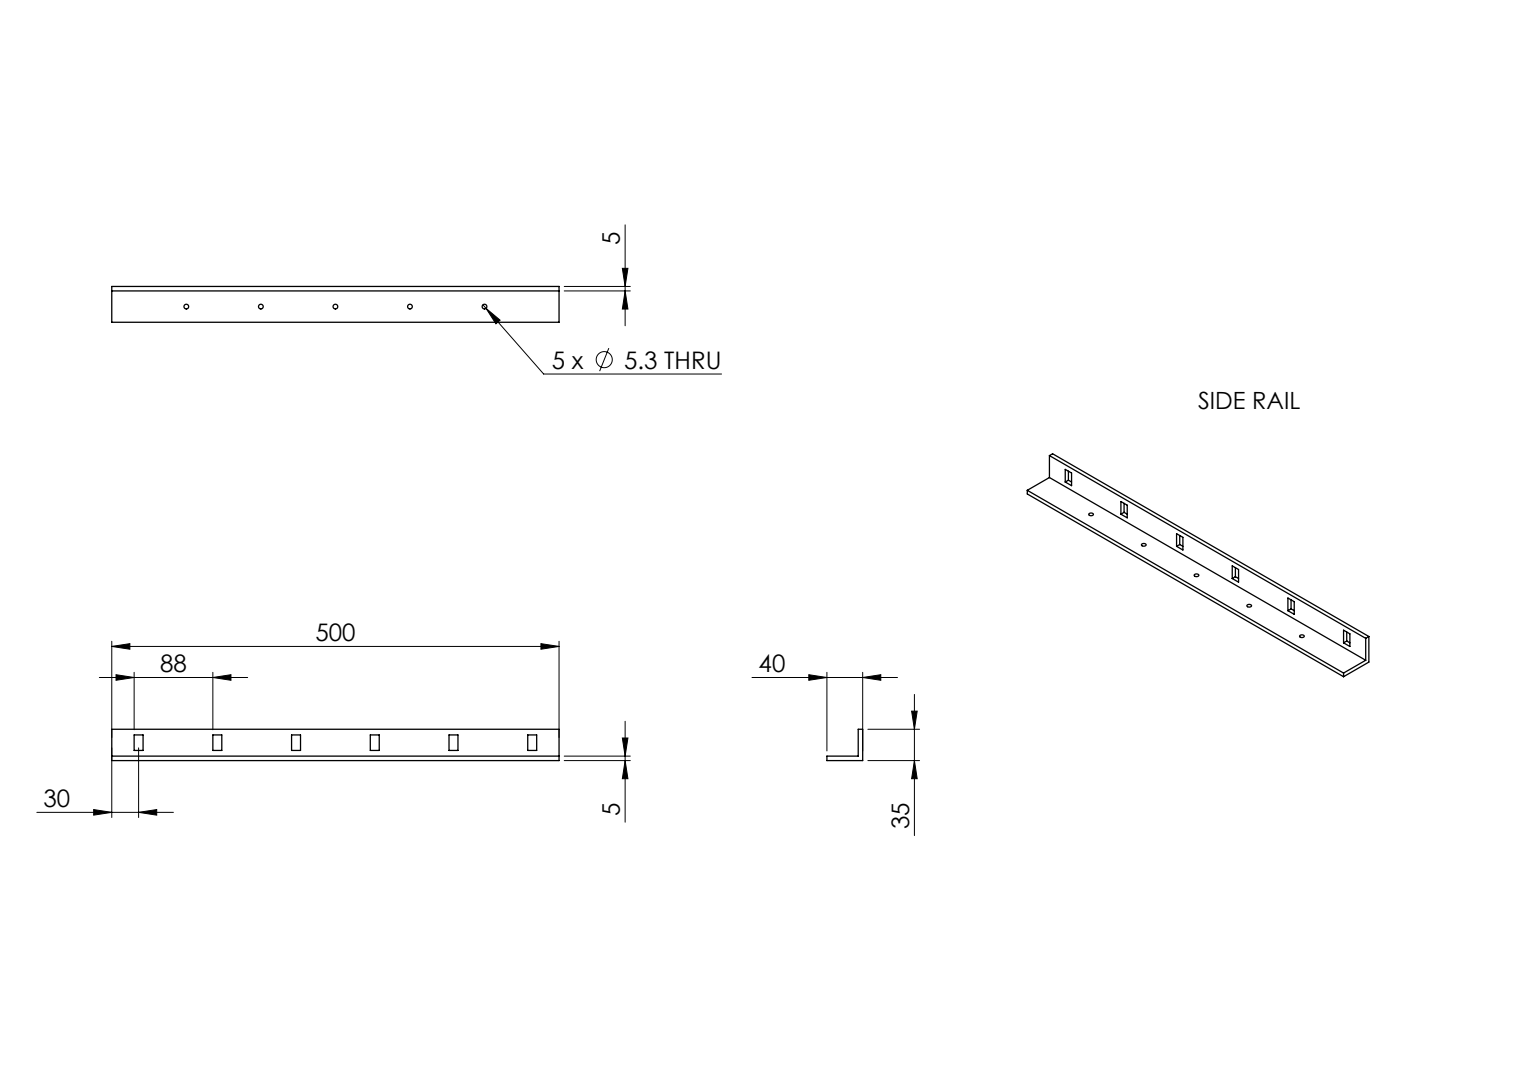
ISO-10303-21;
HEADER;
FILE_DESCRIPTION (('STEP AP214'),
    '1' );
FILE_NAME ('side rail.step',
    '2026-10-24T13:33:06',
    ( '' ),
    ( '' ),
    'SwSTEP 2.0',
    'SolidWorks 2026',
    '' );
FILE_SCHEMA (( 'AUTOMOTIVE_DESIGN' ));
ENDSEC;

DATA;
#21=VECTOR ( 'NONE', #6060, 1000.000000000000000 ) ;
#37=ADVANCED_FACE ( 'NONE', ( #11695 ), #12926, .T. ) ;
#81=ADVANCED_FACE ( 'NONE', ( #7413, #11845, #1899, #419, #4888, #9306, #3544 ), #4372, .T. ) ;
#89=PLANE ( 'NONE',  #11765 ) ;
#114=ORIENTED_EDGE ( 'NONE', *, *, #1574, .F. ) ;
#116=AXIS2_PLACEMENT_3D ( 'NONE', #1990, #12809, #3959 ) ;
#129=CARTESIAN_POINT ( 'NONE',  ( 357.0000000000000000, 8.660254037844390851, 205.0000000000000284 ) ) ;
#143=CARTESIAN_POINT ( 'NONE',  ( 93.00000000000000000, -8.660254037844389075, 199.9990000000000236 ) ) ;
#156=ADVANCED_FACE ( 'NONE', ( #2113 ), #8789, .F. ) ;
#158=CYLINDRICAL_SURFACE ( 'NONE', #4474, 2.649999999999985700 ) ;
#167=EDGE_CURVE ( 'NONE', #11965, #7113, #13067, .T. ) ;
#176=DIRECTION ( 'NONE',  ( -0.000000000000000000, 1.000000000000000000, 0.000000000000000000 ) ) ;
#194=DIRECTION ( 'NONE',  ( 1.000000000000000000, 0.000000000000000000, 0.000000000000000000 ) ) ;
#222=VECTOR ( 'NONE', #1616, 1000.000000000000000 ) ;
#227=FILL_AREA_STYLE ('',( #2582 ) ) ;
#231=LINE ( 'NONE', #7733, #9690 ) ;
#254=DIRECTION ( 'NONE',  ( -1.000000000000000000, 0.000000000000000000, 0.000000000000000000 ) ) ;
#257=ORIENTED_EDGE ( 'NONE', *, *, #9709, .T. ) ;
#259=DIRECTION ( 'NONE',  ( 0.000000000000000000, 0.000000000000000000, 1.000000000000000000 ) ) ;
#261=ORIENTED_EDGE ( 'NONE', *, *, #3754, .T. ) ;
#280=EDGE_LOOP ( 'NONE', ( #548, #583, #6220, #3150 ) ) ;
#285=CARTESIAN_POINT ( 'NONE',  ( 259.0000000000000000, 8.660254037844390851, 205.0000000000000284 ) ) ;
#302=EDGE_CURVE ( 'NONE', #5376, #611, #2399, .T. ) ;
#303=FACE_OUTER_BOUND ( 'NONE', #3913, .T. ) ;
#308=EDGE_CURVE ( 'NONE', #574, #7171, #11477, .T. ) ;
#311=DIRECTION ( 'NONE',  ( -0.000000000000000000, 1.000000000000000000, 0.000000000000000000 ) ) ;
#327=ADVANCED_FACE ( 'NONE', ( #11322 ), #1364, .F. ) ;
#335=DIRECTION ( 'NONE',  ( 0.000000000000000000, 1.000000000000000000, 0.000000000000000000 ) ) ;
#340=EDGE_CURVE ( 'NONE', #10091, #12864, #5804, .T. ) ;
#352=EDGE_LOOP ( 'NONE', ( #7551, #6628 ) ) ;
#359=VECTOR ( 'NONE', #3088, 1000.000000000000000 ) ;
#373=CIRCLE ( 'NONE', #6200, 2.649999999999985700 ) ;
#392=VECTOR ( 'NONE', #9688, 1000.000000000000000 ) ;
#393=DIRECTION ( 'NONE',  ( 0.000000000000000000, 0.000000000000000000, 1.000000000000000000 ) ) ;
#396=ORIENTED_EDGE ( 'NONE', *, *, #10733, .F. ) ;
#397=CARTESIAN_POINT ( 'NONE',  ( 82.99999999999998579, -8.660254037844389075, 200.0000000000000000 ) ) ;
#410=CARTESIAN_POINT ( 'NONE',  ( -30.00000000000002842, 15.00000000000000000, 205.0000000000000284 ) ) ;
#419=FACE_BOUND ( 'NONE', #9154, .T. ) ;
#424=ORIENTED_EDGE ( 'NONE', *, *, #1321, .T. ) ;
#426=ADVANCED_FACE ( 'NONE', ( #13912 ), #3987, .F. ) ;
#427=DIRECTION ( 'NONE',  ( -1.000000000000000000, 0.000000000000000000, 0.000000000000000000 ) ) ;
#441=LINE ( 'NONE', #4910, #14145 ) ;
#471=VECTOR ( 'NONE', #1834, 1000.000000000000000 ) ;
#486=VERTEX_POINT ( 'NONE', #1503 ) ;
#487=FACE_BOUND ( 'NONE', #5303, .T. ) ;
#494=DIRECTION ( 'NONE',  ( -0.000000000000000000, -0.000000000000000000, 1.000000000000000000 ) ) ;
#507=LINE ( 'NONE', #9385, #4377 ) ;
#514=VERTEX_POINT ( 'NONE', #397 ) ;
#515=( LENGTH_UNIT ( ) NAMED_UNIT ( * ) SI_UNIT ( .MILLI., .METRE. ) );
#521=ORIENTED_EDGE ( 'NONE', *, *, #4268, .F. ) ;
#526=VECTOR ( 'NONE', #13201, 1000.000000000000000 ) ;
#532=VERTEX_POINT ( 'NONE', #10807 ) ;
#537=CARTESIAN_POINT ( 'NONE',  ( 347.0000000000000000, 8.660254037844390851, 199.9990000000000236 ) ) ;
#544=AXIS2_PLACEMENT_3D ( 'NONE', #926, #9879, #13212 ) ;
#545=DIRECTION ( 'NONE',  ( 0.000000000000000000, 0.000000000000000000, 1.000000000000000000 ) ) ;
#548=ORIENTED_EDGE ( 'NONE', *, *, #9525, .F. ) ;
#549=DIRECTION ( 'NONE',  ( -1.000000000000000000, 0.000000000000000000, -0.000000000000000000 ) ) ;
#554=DIRECTION ( 'NONE',  ( 0.000000000000000000, 0.000000000000000000, 1.000000000000000000 ) ) ;
#558=ORIENTED_EDGE ( 'NONE', *, *, #6357, .F. ) ;
#559=FACE_BOUND ( 'NONE', #6521, .T. ) ;
#560=ADVANCED_FACE ( 'NONE', ( #13188 ), #11821, .F. ) ;
#574=VERTEX_POINT ( 'NONE', #11897 ) ;
#583=ORIENTED_EDGE ( 'NONE', *, *, #10908, .F. ) ;
#590=LINE ( 'NONE', #1845, #7331 ) ;
#607=CARTESIAN_POINT ( 'NONE',  ( 53.33333333333330017, -20.00000000000000000, 225.1500000000000625 ) ) ;
#611=VERTEX_POINT ( 'NONE', #9793 ) ;
#617=DIRECTION ( 'NONE',  ( -0.000000000000000000, -0.000000000000000000, 1.000000000000000000 ) ) ;
#621=DIRECTION ( 'NONE',  ( -0.000000000000000000, -0.000000000000000000, 1.000000000000000000 ) ) ;
#622=FACE_BOUND ( 'NONE', #8043, .T. ) ;
#629=ORIENTED_EDGE ( 'NONE', *, *, #10325, .T. ) ;
#633=CARTESIAN_POINT ( 'NONE',  ( 386.6666666666666288, -14.99999999999999822, 219.8500000000001080 ) ) ;
#638=EDGE_LOOP ( 'NONE', ( #7545, #6355, #6179, #9350 ) ) ;
#643=ADVANCED_FACE ( 'NONE', ( #9643 ), #839, .F. ) ;
#696=ORIENTED_EDGE ( 'NONE', *, *, #2963, .T. ) ;
#703=PLANE ( 'NONE',  #2931 ) ;
#709=FACE_OUTER_BOUND ( 'NONE', #10738, .T. ) ;
#718=ORIENTED_EDGE ( 'NONE', *, *, #4541, .F. ) ;
#720=EDGE_CURVE ( 'NONE', #10091, #8663, #9863, .T. ) ;
#725=CARTESIAN_POINT ( 'NONE',  ( 259.0000000000000000, 8.660254037844390851, 199.9990000000000236 ) ) ;
#730=DIRECTION ( 'NONE',  ( 1.000000000000000000, 0.000000000000000000, 0.000000000000000000 ) ) ;
#744=ORIENTED_EDGE ( 'NONE', *, *, #9206, .T. ) ;
#769=LINE ( 'NONE', #1579, #4481 ) ;
#784=EDGE_LOOP ( 'NONE', ( #12621, #13135, #7197, #6469 ) ) ;
#788=AXIS2_PLACEMENT_3D ( 'NONE', #10096, #13425, #6557 ) ;
#792=ORIENTED_EDGE ( 'NONE', *, *, #4975, .T. ) ;
#797=CARTESIAN_POINT ( 'NONE',  ( 170.9999999999999716, -8.660254037844389075, 205.0000000000000284 ) ) ;
#806=VERTEX_POINT ( 'NONE', #6663 ) ;
#807=DIRECTION ( 'NONE',  ( 0.000000000000000000, -1.000000000000000000, 0.000000000000000000 ) ) ;
#808=CIRCLE ( 'NONE', #6622, 2.649999999999985700 ) ;
#822=EDGE_LOOP ( 'NONE', ( #3970, #8831, #13317, #6166 ) ) ;
#829=PRODUCT_DEFINITION_CONTEXT ( 'detailed design', #10547, 'design' ) ;
#830=ORIENTED_EDGE ( 'NONE', *, *, #8702, .T. ) ;
#831=DIRECTION ( 'NONE',  ( -0.000000000000000000, 1.000000000000000000, -0.000000000000000000 ) ) ;
#839=PLANE ( 'NONE',  #11489 ) ;
#855=DIRECTION ( 'NONE',  ( 1.000000000000000000, 0.000000000000000000, 0.000000000000000000 ) ) ;
#862=UNCERTAINTY_MEASURE_WITH_UNIT (LENGTH_MEASURE( 1.000000000000000082E-05 ), #515, 'distance_accuracy_value', 'NONE');
#876=AXIS2_PLACEMENT_3D ( 'NONE', #2252, #11112, #2107 ) ;
#898=VERTEX_POINT ( 'NONE', #607 ) ;
#900=EDGE_CURVE ( 'NONE', #7113, #7167, #1368, .T. ) ;
#906=ORIENTED_EDGE ( 'NONE', *, *, #9206, .F. ) ;
#913=FACE_OUTER_BOUND ( 'NONE', #14136, .T. ) ;
#917=CIRCLE ( 'NONE', #12520, 2.649999999999985700 ) ;
#920=FACE_OUTER_BOUND ( 'NONE', #822, .T. ) ;
#925=EDGE_LOOP ( 'NONE', ( #10023, #943, #257, #1375 ) ) ;
#926=CARTESIAN_POINT ( 'NONE',  ( 303.3333333333333144, -15.00000000000000000, 222.5000000000000853 ) ) ;
#930=VERTEX_POINT ( 'NONE', #2815 ) ;
#943=ORIENTED_EDGE ( 'NONE', *, *, #2678, .T. ) ;
#962=CARTESIAN_POINT ( 'NONE',  ( 82.99999999999998579, 8.660254037844390851, 205.0000000000000284 ) ) ;
#964=ORIENTED_EDGE ( 'NONE', *, *, #6331, .T. ) ;
#970=DIRECTION ( 'NONE',  ( 0.000000000000000000, -1.000000000000000000, 0.000000000000000000 ) ) ;
#994=LINE ( 'NONE', #9059, #12994 ) ;
#1021=ORIENTED_EDGE ( 'NONE', *, *, #11142, .T. ) ;
#1041=DIRECTION ( 'NONE',  ( -0.000000000000000000, 1.000000000000000000, 0.000000000000000000 ) ) ;
#1063=DIRECTION ( 'NONE',  ( 0.000000000000000000, 0.000000000000000000, -1.000000000000000000 ) ) ;
#1070=VECTOR ( 'NONE', #2045, 1000.000000000000000 ) ;
#1106=PLANE ( 'NONE',  #10917 ) ;
#1107=LINE ( 'NONE', #5555, #2077 ) ;
#1139=LINE ( 'NONE', #5516, #526 ) ;
#1151=VERTEX_POINT ( 'NONE', #8203 ) ;
#1155=EDGE_CURVE ( 'NONE', #12855, #4614, #1461, .T. ) ;
#1156=EDGE_LOOP ( 'NONE', ( #5436, #9530, #5592, #6967 ) ) ;
#1158=EDGE_LOOP ( 'NONE', ( #6888, #7499, #114, #558 ) ) ;
#1182=CARTESIAN_POINT ( 'NONE',  ( 136.6666666666666288, -20.00000000000000000, 222.5000000000000853 ) ) ;
#1209=ORIENTED_EDGE ( 'NONE', *, *, #1854, .T. ) ;
#1221=EDGE_CURVE ( 'NONE', #8720, #14065, #6982, .T. ) ;
#1227=LINE ( 'NONE', #3497, #6780 ) ;
#1228=ORIENTED_EDGE ( 'NONE', *, *, #5685, .F. ) ;
#1233=DIRECTION ( 'NONE',  ( 0.000000000000000000, 0.000000000000000000, 1.000000000000000000 ) ) ;
#1236=( NAMED_UNIT ( * ) SI_UNIT ( $, .STERADIAN. ) SOLID_ANGLE_UNIT ( ) );
#1250=EDGE_CURVE ( 'NONE', #4587, #12687, #13572, .T. ) ;
#1277=DIRECTION ( 'NONE',  ( 0.000000000000000000, -1.000000000000000000, 0.000000000000000000 ) ) ;
#1308=CARTESIAN_POINT ( 'NONE',  ( 303.3333333333333144, -15.00000000000000000, 225.1500000000000625 ) ) ;
#1321=EDGE_CURVE ( 'NONE', #13567, #5456, #13939, .T. ) ;
#1332=VERTEX_POINT ( 'NONE', #4961 ) ;
#1346=CARTESIAN_POINT ( 'NONE',  ( 386.6666666666666288, -20.00000000000000000, 222.5000000000000853 ) ) ;
#1350=EDGE_CURVE ( 'NONE', #5388, #6497, #3002, .T. ) ;
#1356=FACE_OUTER_BOUND ( 'NONE', #5395, .T. ) ;
#1364=CYLINDRICAL_SURFACE ( 'NONE', #3147, 2.649999999999985700 ) ;
#1366=CARTESIAN_POINT ( 'NONE',  ( 434.9999999999999432, 8.660254037844390851, 199.9990000000000236 ) ) ;
#1368=CIRCLE ( 'NONE', #12741, 2.649999999999985700 ) ;
#1375=ORIENTED_EDGE ( 'NONE', *, *, #13935, .T. ) ;
#1393=VECTOR ( 'NONE', #7157, 1000.000000000000000 ) ;
#1423=EDGE_LOOP ( 'NONE', ( #8180, #5861, #11249, #6169 ) ) ;
#1426=CARTESIAN_POINT ( 'NONE',  ( 434.9999999999999432, -8.660254037844389075, 199.9990000000000236 ) ) ;
#1445=VECTOR ( 'NONE', #3310, 1000.000000000000000 ) ;
#1461=LINE ( 'NONE', #5971, #12295 ) ;
#1462=EDGE_LOOP ( 'NONE', ( #7055, #3073, #3390, #9366, #2015, #2649 ) ) ;
#1472=ORIENTED_EDGE ( 'NONE', *, *, #302, .F. ) ;
#1476=CARTESIAN_POINT ( 'NONE',  ( 181.0000000000000000, 8.660254037844390851, 200.0000000000000000 ) ) ;
#1496=ADVANCED_FACE ( 'NONE', ( #10029 ), #9955, .F. ) ;
#1500=ORIENTED_EDGE ( 'NONE', *, *, #7562, .F. ) ;
#1503=CARTESIAN_POINT ( 'NONE',  ( 93.00000000000000000, 8.660254037844390851, 200.0000000000000000 ) ) ;
#1511=DIRECTION ( 'NONE',  ( 1.000000000000000000, 0.000000000000000000, 0.000000000000000000 ) ) ;
#1521=VECTOR ( 'NONE', #4856, 1000.000000000000000 ) ;
#1525=EDGE_LOOP ( 'NONE', ( #12096, #1587 ) ) ;
#1533=ORIENTED_EDGE ( 'NONE', *, *, #302, .T. ) ;
#1534=CARTESIAN_POINT ( 'NONE',  ( -5.000000000000000888, 8.660254037844390851, 205.0000000000000284 ) ) ;
#1543=VECTOR ( 'NONE', #13285, 1000.000000000000000 ) ;
#1544=ORIENTED_EDGE ( 'NONE', *, *, #720, .F. ) ;
#1547=DIRECTION ( 'NONE',  ( 0.000000000000000000, 0.000000000000000000, 1.000000000000000000 ) ) ;
#1553=EDGE_CURVE ( 'NONE', #8456, #8038, #4796, .T. ) ;
#1574=EDGE_CURVE ( 'NONE', #3366, #4058, #6753, .T. ) ;
#1576=EDGE_CURVE ( 'NONE', #8786, #486, #1227, .T. ) ;
#1579=CARTESIAN_POINT ( 'NONE',  ( 470.0000000000000000, 15.00000000000000000, 205.0000000000000284 ) ) ;
#1586=DIRECTION ( 'NONE',  ( 1.000000000000000000, 0.000000000000000000, 0.000000000000000000 ) ) ;
#1587=ORIENTED_EDGE ( 'NONE', *, *, #6484, .T. ) ;
#1590=CARTESIAN_POINT ( 'NONE',  ( 259.0000000000000000, -8.660254037844389075, 200.0000000000000000 ) ) ;
#1606=LINE ( 'NONE', #4020, #8260 ) ;
#1616=DIRECTION ( 'NONE',  ( 0.000000000000000000, 1.000000000000000000, 0.000000000000000000 ) ) ;
#1650=ORIENTED_EDGE ( 'NONE', *, *, #13490, .T. ) ;
#1659=CARTESIAN_POINT ( 'NONE',  ( 136.6666666666666288, -14.99999999999999822, 219.8500000000001080 ) ) ;
#1661=VECTOR ( 'NONE', #6856, 1000.000000000000000 ) ;
#1673=EDGE_LOOP ( 'NONE', ( #9501, #13329, #5600, #2944 ) ) ;
#1675=CIRCLE ( 'NONE', #11651, 2.649999999999985700 ) ;
#1692=ORIENTED_EDGE ( 'NONE', *, *, #11438, .T. ) ;
#1698=ORIENTED_EDGE ( 'NONE', *, *, #11906, .T. ) ;
#1712=DIRECTION ( 'NONE',  ( 0.000000000000000000, -0.000000000000000000, -1.000000000000000000 ) ) ;
#1715=CARTESIAN_POINT ( 'NONE',  ( 434.9999999999999432, -8.660254037844389075, 205.0000000000000284 ) ) ;
#1732=CARTESIAN_POINT ( 'NONE',  ( 269.0000000000000000, -8.660254037844389075, 200.0000000000000000 ) ) ;
#1746=CARTESIAN_POINT ( 'NONE',  ( 269.0000000000000000, 8.660254037844390851, 205.0000000000000284 ) ) ;
#1757=CIRCLE ( 'NONE', #14043, 2.649999999999985700 ) ;
#1760=ADVANCED_BREP_SHAPE_REPRESENTATION ( '', ( #3714, #14039 ), #3087 ) ;
#1772=VECTOR ( 'NONE', #10843, 1000.000000000000000 ) ;
#1779=LINE ( 'NONE', #8531, #7857 ) ;
#1789=DIRECTION ( 'NONE',  ( -0.000000000000000000, -0.000000000000000000, 1.000000000000000000 ) ) ;
#1794=AXIS2_PLACEMENT_3D ( 'NONE', #11740, #10875, #9715 ) ;
#1797=EDGE_CURVE ( 'NONE', #2838, #12140, #769, .T. ) ;
#1822=EDGE_LOOP ( 'NONE', ( #13493, #1021, #5094, #2101 ) ) ;
#1834=DIRECTION ( 'NONE',  ( 0.000000000000000000, 1.000000000000000000, 0.000000000000000000 ) ) ;
#1844=ORIENTED_EDGE ( 'NONE', *, *, #1574, .T. ) ;
#1845=CARTESIAN_POINT ( 'NONE',  ( 434.9999999999999432, -8.660254037844389075, 200.0000000000000000 ) ) ;
#1854=EDGE_CURVE ( 'NONE', #8482, #10176, #4060, .T. ) ;
#1873=CARTESIAN_POINT ( 'NONE',  ( 93.00000000000000000, 8.660254037844390851, 199.9990000000000236 ) ) ;
#1884=ORIENTED_EDGE ( 'NONE', *, *, #9683, .T. ) ;
#1897=EDGE_CURVE ( 'NONE', #532, #10192, #9273, .T. ) ;
#1899=FACE_OUTER_BOUND ( 'NONE', #4056, .T. ) ;
#1909=CARTESIAN_POINT ( 'NONE',  ( -30.00000000000002842, -20.00000000000000000, 200.0000000000000000 ) ) ;
#1921=CARTESIAN_POINT ( 'NONE',  ( 136.6666666666666288, -20.00000000000000000, 225.1500000000000625 ) ) ;
#1930=ADVANCED_FACE ( 'NONE', ( #8772 ), #14063, .F. ) ;
#1938=PLANE ( 'NONE',  #1794 ) ;
#1939=DIRECTION ( 'NONE',  ( -1.000000000000000000, 0.000000000000000000, -0.000000000000000000 ) ) ;
#1949=ORIENTED_EDGE ( 'NONE', *, *, #11119, .T. ) ;
#1952=CARTESIAN_POINT ( 'NONE',  ( 170.9999999999999716, 8.660254037844390851, 199.9990000000000236 ) ) ;
#1957=DIRECTION ( 'NONE',  ( 1.000000000000000000, 0.000000000000000000, 0.000000000000000000 ) ) ;
#1990=CARTESIAN_POINT ( 'NONE',  ( 303.3333333333333144, -20.00000000000000000, 222.5000000000000853 ) ) ;
#1994=AXIS2_PLACEMENT_3D ( 'NONE', #3763, #10431, #6004 ) ;
#2015=ORIENTED_EDGE ( 'NONE', *, *, #9683, .F. ) ;
#2040=DIRECTION ( 'NONE',  ( -0.000000000000000000, 1.000000000000000000, 0.000000000000000000 ) ) ;
#2041=UNCERTAINTY_MEASURE_WITH_UNIT (LENGTH_MEASURE( 1.000000000000000082E-05 ), #8000, 'distance_accuracy_value', 'NONE');
#2045=DIRECTION ( 'NONE',  ( -0.000000000000000000, -0.000000000000000000, 1.000000000000000000 ) ) ;
#2047=CARTESIAN_POINT ( 'NONE',  ( 170.9999999999999716, 8.660254037844390851, 200.0000000000000000 ) ) ;
#2056=DIRECTION ( 'NONE',  ( 0.000000000000000000, 0.000000000000000000, 1.000000000000000000 ) ) ;
#2059=EDGE_LOOP ( 'NONE', ( #13294, #3495, #8438, #8654 ) ) ;
#2060=LINE ( 'NONE', #6629, #1445 ) ;
#2077=VECTOR ( 'NONE', #14177, 1000.000000000000000 ) ;
#2089=EDGE_CURVE ( 'NONE', #6981, #8456, #1779, .T. ) ;
#2101=ORIENTED_EDGE ( 'NONE', *, *, #4096, .F. ) ;
#2107=DIRECTION ( 'NONE',  ( 0.000000000000000000, 0.000000000000000000, 1.000000000000000000 ) ) ;
#2113=FACE_OUTER_BOUND ( 'NONE', #6177, .T. ) ;
#2116=VECTOR ( 'NONE', #855, 1000.000000000000000 ) ;
#2127=LINE ( 'NONE', #5400, #1772 ) ;
#2163=EDGE_CURVE ( 'NONE', #10673, #5456, #2738, .T. ) ;
#2188=DIRECTION ( 'NONE',  ( 0.000000000000000000, -0.000000000000000000, 1.000000000000000000 ) ) ;
#2219=DIRECTION ( 'NONE',  ( 1.000000000000000000, 0.000000000000000000, 0.000000000000000000 ) ) ;
#2221=FACE_BOUND ( 'NONE', #2786, .T. ) ;
#2240=FACE_OUTER_BOUND ( 'NONE', #13467, .T. ) ;
#2252=CARTESIAN_POINT ( 'NONE',  ( 303.3333333333333144, -15.00000000000000000, 222.5000000000000853 ) ) ;
#2254=VECTOR ( 'NONE', #9603, 1000.000000000000000 ) ;
#2268=CIRCLE ( 'NONE', #6202, 2.649999999999985700 ) ;
#2283=FACE_OUTER_BOUND ( 'NONE', #2836, .T. ) ;
#2308=ORIENTED_EDGE ( 'NONE', *, *, #13568, .T. ) ;
#2327=VERTEX_POINT ( 'NONE', #962 ) ;
#2331=VECTOR ( 'NONE', #3546, 1000.000000000000000 ) ;
#2334=EDGE_CURVE ( 'NONE', #2529, #12855, #12370, .T. ) ;
#2340=CARTESIAN_POINT ( 'NONE',  ( 470.0000000000000000, 0.000000000000000000, 205.0000000000000284 ) ) ;
#2356=DIRECTION ( 'NONE',  ( 0.000000000000000000, -0.000000000000000000, -1.000000000000000000 ) ) ;
#2361=LINE ( 'NONE', #11077, #11596 ) ;
#2368=CARTESIAN_POINT ( 'NONE',  ( 303.3333333333333144, -20.00000000000000000, 225.1500000000000625 ) ) ;
#2369=DIRECTION ( 'NONE',  ( 0.000000000000000000, 0.000000000000000000, 1.000000000000000000 ) ) ;
#2371=DIRECTION ( 'NONE',  ( -1.000000000000000000, 0.000000000000000000, 0.000000000000000000 ) ) ;
#2399=LINE ( 'NONE', #4512, #13534 ) ;
#2419=DIRECTION ( 'NONE',  ( -1.000000000000000000, 0.000000000000000000, -0.000000000000000000 ) ) ;
#2425=CLOSED_SHELL ( 'NONE', ( #10182, #6516, #327, #4010, #2688, #6499, #8614, #3759, #10923, #6035, #2848, #7603, #6053, #7191, #13852, #1496, #1930, #11232, #426, #7203, #10827, #643, #7016, #8801, #4439, #81, #37, #8347, #12972, #3378, #9001, #2795, #9488, #5963, #13581, #560, #7381, #9658, #156, #7500, #3144, #4173 ) ) ;
#2435=CARTESIAN_POINT ( 'NONE',  ( 444.9999999999999432, 8.660254037844390851, 200.0000000000000000 ) ) ;
#2440=LINE ( 'NONE', #9038, #8558 ) ;
#2464=VERTEX_POINT ( 'NONE', #4385 ) ;
#2473=EDGE_LOOP ( 'NONE', ( #13133, #1209, #9047, #6416 ) ) ;
#2476=CIRCLE ( 'NONE', #12423, 2.649999999999985700 ) ;
#2498=FACE_OUTER_BOUND ( 'NONE', #2653, .T. ) ;
#2509=ORIENTED_EDGE ( 'NONE', *, *, #13670, .T. ) ;
#2511=EDGE_CURVE ( 'NONE', #6112, #8606, #7297, .T. ) ;
#2517=VERTEX_POINT ( 'NONE', #4523 ) ;
#2529=VERTEX_POINT ( 'NONE', #129 ) ;
#2532=CARTESIAN_POINT ( 'NONE',  ( 53.33333333333330017, -14.99999999999999822, 225.1500000000000625 ) ) ;
#2538=DIRECTION ( 'NONE',  ( -0.000000000000000000, 1.000000000000000000, -0.000000000000000000 ) ) ;
#2551=FACE_OUTER_BOUND ( 'NONE', #6774, .T. ) ;
#2571=LINE ( 'NONE', #11559, #11541 ) ;
#2574=DIRECTION ( 'NONE',  ( 0.000000000000000000, -1.000000000000000000, 0.000000000000000000 ) ) ;
#2582=FILL_AREA_STYLE_COLOUR ( '', #12333 ) ;
#2584=CARTESIAN_POINT ( 'NONE',  ( 170.9999999999999716, 8.660254037844390851, 200.0000000000000000 ) ) ;
#2587=VECTOR ( 'NONE', #2574, 1000.000000000000000 ) ;
#2601=ORIENTED_EDGE ( 'NONE', *, *, #10191, .F. ) ;
#2607=DIRECTION ( 'NONE',  ( -0.000000000000000000, 1.000000000000000000, -0.000000000000000000 ) ) ;
#2637=EDGE_CURVE ( 'NONE', #3406, #1151, #10240, .T. ) ;
#2645=LINE ( 'NONE', #10327, #222 ) ;
#2649=ORIENTED_EDGE ( 'NONE', *, *, #4541, .T. ) ;
#2653=EDGE_LOOP ( 'NONE', ( #10031, #6056, #2509, #8651 ) ) ;
#2655=EDGE_CURVE ( 'NONE', #1332, #9383, #10399, .T. ) ;
#2659=DIRECTION ( 'NONE',  ( 0.000000000000000000, 1.000000000000000000, 0.000000000000000000 ) ) ;
#2664=LINE ( 'NONE', #5858, #6505 ) ;
#2678=EDGE_CURVE ( 'NONE', #9294, #7034, #4737, .T. ) ;
#2688=ADVANCED_FACE ( 'NONE', ( #11544 ), #10169, .F. ) ;
#2695=LINE ( 'NONE', #11472, #7591 ) ;
#2728=CIRCLE ( 'NONE', #8975, 2.649999999999985700 ) ;
#2738=LINE ( 'NONE', #13818, #8565 ) ;
#2739=DIRECTION ( 'NONE',  ( -0.000000000000000000, 0.000000000000000000, 1.000000000000000000 ) ) ;
#2742=VECTOR ( 'NONE', #3889, 1000.000000000000000 ) ;
#2756=CARTESIAN_POINT ( 'NONE',  ( 170.9999999999999716, 8.660254037844390851, 199.9990000000000236 ) ) ;
#2786=EDGE_LOOP ( 'NONE', ( #13164, #6145 ) ) ;
#2795=ADVANCED_FACE ( 'NONE', ( #6173 ), #4070, .F. ) ;
#2812=CARTESIAN_POINT ( 'NONE',  ( 259.0000000000000000, 8.660254037844390851, 205.0000000000000284 ) ) ;
#2815=CARTESIAN_POINT ( 'NONE',  ( 444.9999999999999432, 8.660254037844390851, 200.0000000000000000 ) ) ;
#2816=DIRECTION ( 'NONE',  ( 0.000000000000000000, -1.000000000000000000, 0.000000000000000000 ) ) ;
#2835=DIRECTION ( 'NONE',  ( -0.000000000000000000, -0.000000000000000000, -1.000000000000000000 ) ) ;
#2836=EDGE_LOOP ( 'NONE', ( #13020, #830, #4442, #5052 ) ) ;
#2838=VERTEX_POINT ( 'NONE', #10680 ) ;
#2842=VERTEX_POINT ( 'NONE', #2844 ) ;
#2844=CARTESIAN_POINT ( 'NONE',  ( 303.3333333333333144, -14.99999999999999822, 225.1500000000000625 ) ) ;
#2848=ADVANCED_FACE ( 'NONE', ( #709 ), #12919, .F. ) ;
#2849=SHAPE_DEFINITION_REPRESENTATION ( #7724, #3832 ) ;
#2856=ORIENTED_EDGE ( 'NONE', *, *, #11438, .F. ) ;
#2860=LINE ( 'NONE', #7697, #1070 ) ;
#2868=DIRECTION ( 'NONE',  ( -0.000000000000000000, 1.000000000000000000, -0.000000000000000000 ) ) ;
#2876=LINE ( 'NONE', #9695, #5702 ) ;
#2880=ORIENTED_EDGE ( 'NONE', *, *, #8265, .T. ) ;
#2916=CARTESIAN_POINT ( 'NONE',  ( 444.9999999999999432, -8.660254037844389075, 205.0000000000000284 ) ) ;
#2917=VECTOR ( 'NONE', #10839, 1000.000000000000000 ) ;
#2921=ORIENTED_EDGE ( 'NONE', *, *, #14198, .F. ) ;
#2931=AXIS2_PLACEMENT_3D ( 'NONE', #7474, #14068, #9653 ) ;
#2944=ORIENTED_EDGE ( 'NONE', *, *, #6357, .T. ) ;
#2945=CARTESIAN_POINT ( 'NONE',  ( 181.0000000000000000, 8.660254037844390851, 205.0000000000000284 ) ) ;
#2950=VECTOR ( 'NONE', #254, 1000.000000000000000 ) ;
#2952=VECTOR ( 'NONE', #10305, 1000.000000000000000 ) ;
#2961=ORIENTED_EDGE ( 'NONE', *, *, #3232, .T. ) ;
#2963=EDGE_CURVE ( 'NONE', #10177, #10192, #1139, .T. ) ;
#2964=ORIENTED_EDGE ( 'NONE', *, *, #900, .F. ) ;
#2975=LINE ( 'NONE', #12897, #5543 ) ;
#2995=CARTESIAN_POINT ( 'NONE',  ( 347.0000000000000000, -8.660254037844389075, 205.0000000000000284 ) ) ;
#2999=ORIENTED_EDGE ( 'NONE', *, *, #3883, .F. ) ;
#3000=DIRECTION ( 'NONE',  ( 1.000000000000000000, 0.000000000000000000, 0.000000000000000000 ) ) ;
#3002=LINE ( 'NONE', #1746, #6306 ) ;
#3004=ORIENTED_EDGE ( 'NONE', *, *, #3830, .T. ) ;
#3015=LINE ( 'NONE', #7210, #392 ) ;
#3020=DIRECTION ( 'NONE',  ( 0.000000000000000000, 1.000000000000000000, 0.000000000000000000 ) ) ;
#3043=EDGE_CURVE ( 'NONE', #6309, #12855, #994, .T. ) ;
#3073=ORIENTED_EDGE ( 'NONE', *, *, #1797, .F. ) ;
#3087=( GEOMETRIC_REPRESENTATION_CONTEXT ( 3 ) GLOBAL_UNCERTAINTY_ASSIGNED_CONTEXT ( ( #862 ) ) GLOBAL_UNIT_ASSIGNED_CONTEXT ( ( #515, #3884, #12372 ) ) REPRESENTATION_CONTEXT ( 'NONE', 'WORKASPACE' ) );
#3088=DIRECTION ( 'NONE',  ( -0.000000000000000000, -0.000000000000000000, 1.000000000000000000 ) ) ;
#3089=VECTOR ( 'NONE', #9000, 1000.000000000000000 ) ;
#3092=CARTESIAN_POINT ( 'NONE',  ( 53.33333333333330017, -20.00000000000000000, 222.5000000000000853 ) ) ;
#3103=VECTOR ( 'NONE', #5011, 1000.000000000000000 ) ;
#3136=ORIENTED_EDGE ( 'NONE', *, *, #10935, .F. ) ;
#3144=ADVANCED_FACE ( 'NONE', ( #11315 ), #12605, .F. ) ;
#3147=AXIS2_PLACEMENT_3D ( 'NONE', #5594, #13624, #259 ) ;
#3150=ORIENTED_EDGE ( 'NONE', *, *, #8702, .F. ) ;
#3153=CARTESIAN_POINT ( 'NONE',  ( 259.0000000000000000, 8.660254037844390851, 199.9990000000000236 ) ) ;
#3155=ORIENTED_EDGE ( 'NONE', *, *, #13229, .F. ) ;
#3163=ORIENTED_EDGE ( 'NONE', *, *, #1155, .T. ) ;
#3181=ORIENTED_EDGE ( 'NONE', *, *, #10705, .F. ) ;
#3185=AXIS2_PLACEMENT_3D ( 'NONE', #9924, #1041, #4417 ) ;
#3191=CARTESIAN_POINT ( 'NONE',  ( 259.0000000000000000, 8.660254037844390851, 205.0000000000000284 ) ) ;
#3208=DIRECTION ( 'NONE',  ( 0.000000000000000000, 1.000000000000000000, 0.000000000000000000 ) ) ;
#3209=EDGE_LOOP ( 'NONE', ( #1844, #11234, #8717, #13805 ) ) ;
#3210=CARTESIAN_POINT ( 'NONE',  ( 347.0000000000000000, -8.660254037844389075, 200.0000000000000000 ) ) ;
#3232=EDGE_CURVE ( 'NONE', #8663, #10091, #917, .T. ) ;
#3249=LINE ( 'NONE', #13375, #9928 ) ;
#3262=CARTESIAN_POINT ( 'NONE',  ( -30.00000000000002842, -20.00000000000000000, 200.0000000000000000 ) ) ;
#3280=CARTESIAN_POINT ( 'NONE',  ( 386.6666666666666288, -15.00000000000000000, 222.5000000000000853 ) ) ;
#3307=ORIENTED_EDGE ( 'NONE', *, *, #5685, .T. ) ;
#3310=DIRECTION ( 'NONE',  ( 0.000000000000000000, 1.000000000000000000, 0.000000000000000000 ) ) ;
#3329=EDGE_CURVE ( 'NONE', #5679, #2529, #2361, .T. ) ;
#3335=ORIENTED_EDGE ( 'NONE', *, *, #3232, .F. ) ;
#3350=ORIENTED_EDGE ( 'NONE', *, *, #3883, .T. ) ;
#3366=VERTEX_POINT ( 'NONE', #7858 ) ;
#3378=ADVANCED_FACE ( 'NONE', ( #4476 ), #1106, .F. ) ;
#3387=CARTESIAN_POINT ( 'NONE',  ( -30.00000000000002842, 15.00000000000000000, 205.0000000000000284 ) ) ;
#3390=ORIENTED_EDGE ( 'NONE', *, *, #11119, .F. ) ;
#3396=ORIENTED_EDGE ( 'NONE', *, *, #13670, .F. ) ;
#3405=CIRCLE ( 'NONE', #9410, 2.649999999999985700 ) ;
#3406=VERTEX_POINT ( 'NONE', #3387 ) ;
#3407=VECTOR ( 'NONE', #617, 1000.000000000000000 ) ;
#3413=ORIENTED_EDGE ( 'NONE', *, *, #6989, .T. ) ;
#3415=DIRECTION ( 'NONE',  ( 0.000000000000000000, -0.000000000000000000, -1.000000000000000000 ) ) ;
#3417=VECTOR ( 'NONE', #9163, 1000.000000000000000 ) ;
#3429=DIRECTION ( 'NONE',  ( -0.000000000000000000, 1.000000000000000000, -0.000000000000000000 ) ) ;
#3431=ORIENTED_EDGE ( 'NONE', *, *, #720, .T. ) ;
#3485=EDGE_CURVE ( 'NONE', #10176, #13937, #2645, .T. ) ;
#3495=ORIENTED_EDGE ( 'NONE', *, *, #3576, .T. ) ;
#3497=CARTESIAN_POINT ( 'NONE',  ( 93.00000000000000000, 8.660254037844390851, 200.0000000000000000 ) ) ;
#3516=FACE_OUTER_BOUND ( 'NONE', #6090, .T. ) ;
#3533=FACE_BOUND ( 'NONE', #9400, .T. ) ;
#3544=FACE_BOUND ( 'NONE', #1673, .T. ) ;
#3546=DIRECTION ( 'NONE',  ( -1.000000000000000000, -0.000000000000000000, -0.000000000000000000 ) ) ;
#3553=CARTESIAN_POINT ( 'NONE',  ( 444.9999999999999432, 8.660254037844390851, 199.9990000000000236 ) ) ;
#3576=EDGE_CURVE ( 'NONE', #7514, #2464, #7350, .T. ) ;
#3579=ORIENTED_EDGE ( 'NONE', *, *, #3749, .F. ) ;
#3582=VERTEX_POINT ( 'NONE', #9686 ) ;
#3608=ORIENTED_EDGE ( 'NONE', *, *, #12502, .F. ) ;
#3609=LINE ( 'NONE', #5576, #13441 ) ;
#3611=ORIENTED_EDGE ( 'NONE', *, *, #2334, .T. ) ;
#3635=CARTESIAN_POINT ( 'NONE',  ( -30.00000000000002842, -15.00000000000000000, 205.0000000000000284 ) ) ;
#3651=CARTESIAN_POINT ( 'NONE',  ( -30.00000000000002842, -20.00000000000000000, 200.0000000000000000 ) ) ;
#3657=CARTESIAN_POINT ( 'NONE',  ( -5.000000000000000888, -8.660254037844389075, 199.9990000000000236 ) ) ;
#3669=SURFACE_STYLE_USAGE ( .BOTH. , #4692 ) ;
#3675=ORIENTED_EDGE ( 'NONE', *, *, #12601, .T. ) ;
#3681=FACE_OUTER_BOUND ( 'NONE', #10157, .T. ) ;
#3704=ORIENTED_EDGE ( 'NONE', *, *, #4998, .T. ) ;
#3714=MANIFOLD_SOLID_BREP ( 'M5 Clearance Hole1', #2425 ) ;
#3722=EDGE_LOOP ( 'NONE', ( #7661, #13068, #6269, #1884 ) ) ;
#3726=CARTESIAN_POINT ( 'NONE',  ( 181.0000000000000000, 8.660254037844390851, 200.0000000000000000 ) ) ;
#3729=VECTOR ( 'NONE', #4243, 1000.000000000000000 ) ;
#3734=VERTEX_POINT ( 'NONE', #8943 ) ;
#3749=EDGE_CURVE ( 'NONE', #11189, #9294, #5931, .T. ) ;
#3754=EDGE_CURVE ( 'NONE', #11555, #2842, #12350, .T. ) ;
#3757=CIRCLE ( 'NONE', #9562, 2.649999999999985700 ) ;
#3759=ADVANCED_FACE ( 'NONE', ( #4310 ), #13153, .F. ) ;
#3763=CARTESIAN_POINT ( 'NONE',  ( 219.9999999999999716, -15.00000000000000000, 222.5000000000000853 ) ) ;
#3767=CARTESIAN_POINT ( 'NONE',  ( 347.0000000000000000, 8.660254037844390851, 200.0000000000000000 ) ) ;
#3788=CARTESIAN_POINT ( 'NONE',  ( 219.9999999999999716, -20.00000000000000000, 222.5000000000000853 ) ) ;
#3796=ORIENTED_EDGE ( 'NONE', *, *, #6767, .F. ) ;
#3797=DIRECTION ( 'NONE',  ( 1.000000000000000000, 0.000000000000000000, 0.000000000000000000 ) ) ;
#3812=ORIENTED_EDGE ( 'NONE', *, *, #11890, .T. ) ;
#3829=LINE ( 'NONE', #6006, #3407 ) ;
#3830=EDGE_CURVE ( 'NONE', #3844, #5376, #4955, .T. ) ;
#3832=SHAPE_REPRESENTATION ( 'side rail', ( #14039 ), #3087 ) ;
#3840=DIRECTION ( 'NONE',  ( -0.000000000000000000, 0.000000000000000000, 1.000000000000000000 ) ) ;
#3844=VERTEX_POINT ( 'NONE', #8275 ) ;
#3861=EDGE_LOOP ( 'NONE', ( #13502, #1650, #12377, #6158 ) ) ;
#3879=VECTOR ( 'NONE', #11827, 1000.000000000000000 ) ;
#3881=AXIS2_PLACEMENT_3D ( 'NONE', #5954, #1586, #4735 ) ;
#3883=EDGE_CURVE ( 'NONE', #4614, #5679, #12996, .T. ) ;
#3884=( NAMED_UNIT ( * ) PLANE_ANGLE_UNIT ( ) SI_UNIT ( $, .RADIAN. ) );
#3887=CARTESIAN_POINT ( 'NONE',  ( 170.9999999999999716, 8.660254037844390851, 205.0000000000000284 ) ) ;
#3889=DIRECTION ( 'NONE',  ( 0.000000000000000000, 1.000000000000000000, 0.000000000000000000 ) ) ;
#3897=DIRECTION ( 'NONE',  ( -0.000000000000000000, 1.000000000000000000, -0.000000000000000000 ) ) ;
#3903=CARTESIAN_POINT ( 'NONE',  ( -30.00000000000000000, 0.000000000000000000, 200.0000000000000000 ) ) ;
#3910=CARTESIAN_POINT ( 'NONE',  ( 170.9999999999999716, 8.660254037844390851, 205.0000000000000284 ) ) ;
#3913=EDGE_LOOP ( 'NONE', ( #10279, #3163, #3608, #6475 ) ) ;
#3929=FACE_BOUND ( 'NONE', #7921, .T. ) ;
#3959=DIRECTION ( 'NONE',  ( 0.000000000000000000, 0.000000000000000000, 1.000000000000000000 ) ) ;
#3970=ORIENTED_EDGE ( 'NONE', *, *, #11906, .F. ) ;
#3982=FACE_BOUND ( 'NONE', #280, .T. ) ;
#3987=PLANE ( 'NONE',  #12167 ) ;
#4010=ADVANCED_FACE ( 'NONE', ( #920 ), #6681, .F. ) ;
#4011=ORIENTED_EDGE ( 'NONE', *, *, #13229, .T. ) ;
#4020=CARTESIAN_POINT ( 'NONE',  ( -5.000000000000000888, 8.660254037844390851, 205.0000000000000284 ) ) ;
#4031=CARTESIAN_POINT ( 'NONE',  ( 303.3333333333333144, -14.99999999999999822, 219.8500000000001080 ) ) ;
#4034=LINE ( 'NONE', #11573, #21 ) ;
#4056=EDGE_LOOP ( 'NONE', ( #1500, #8864, #14071, #10292 ) ) ;
#4058=VERTEX_POINT ( 'NONE', #12056 ) ;
#4060=LINE ( 'NONE', #7104, #12286 ) ;
#4070=PLANE ( 'NONE',  #4934 ) ;
#4081=VERTEX_POINT ( 'NONE', #4291 ) ;
#4086=LINE ( 'NONE', #1909, #11314 ) ;
#4096=EDGE_CURVE ( 'NONE', #486, #13503, #8993, .T. ) ;
#4103=LINE ( 'NONE', #7362, #8988 ) ;
#4137=CARTESIAN_POINT ( 'NONE',  ( 259.0000000000000000, 8.660254037844390851, 199.9990000000000236 ) ) ;
#4152=APPLICATION_CONTEXT ( 'automotive_design' ) ;
#4162=PLANE ( 'NONE',  #8969 ) ;
#4163=CARTESIAN_POINT ( 'NONE',  ( -5.000000000000000888, 8.660254037844390851, 199.9990000000000236 ) ) ;
#4173=ADVANCED_FACE ( 'NONE', ( #5724 ), #11454, .F. ) ;
#4237=EDGE_LOOP ( 'NONE', ( #6549, #792, #4293, #906 ) ) ;
#4243=DIRECTION ( 'NONE',  ( 1.000000000000000000, 0.000000000000000000, 0.000000000000000000 ) ) ;
#4254=VECTOR ( 'NONE', #8256, 1000.000000000000000 ) ;
#4265=LINE ( 'NONE', #13036, #11147 ) ;
#4268=EDGE_CURVE ( 'NONE', #9383, #1332, #9944, .T. ) ;
#4291=CARTESIAN_POINT ( 'NONE',  ( 444.9999999999999432, -8.660254037844389075, 200.0000000000000000 ) ) ;
#4293=ORIENTED_EDGE ( 'NONE', *, *, #2511, .T. ) ;
#4310=FACE_OUTER_BOUND ( 'NONE', #1158, .T. ) ;
#4316=VERTEX_POINT ( 'NONE', #14120 ) ;
#4353=EDGE_CURVE ( 'NONE', #930, #4652, #2975, .T. ) ;
#4360=AXIS2_PLACEMENT_3D ( 'NONE', #3553, #12391, #1063 ) ;
#4372=PLANE ( 'NONE',  #9620 ) ;
#4375=EDGE_CURVE ( 'NONE', #10192, #13567, #7309, .T. ) ;
#4377=VECTOR ( 'NONE', #8289, 1000.000000000000000 ) ;
#4382=PRODUCT ( 'side rail', 'side rail', '', ( #4884 ) ) ;
#4383=CARTESIAN_POINT ( 'NONE',  ( 136.6666666666666288, -14.99999999999999822, 222.5000000000000853 ) ) ;
#4385=CARTESIAN_POINT ( 'NONE',  ( 4.999999999999999112, -8.660254037844389075, 200.0000000000000000 ) ) ;
#4406=DIRECTION ( 'NONE',  ( -0.000000000000000000, 1.000000000000000000, -0.000000000000000000 ) ) ;
#4413=( GEOMETRIC_REPRESENTATION_CONTEXT ( 3 ) GLOBAL_UNCERTAINTY_ASSIGNED_CONTEXT ( ( #8507 ) ) GLOBAL_UNIT_ASSIGNED_CONTEXT ( ( #6830, #9894, #1236 ) ) REPRESENTATION_CONTEXT ( 'NONE', 'WORKASPACE' ) );
#4417=DIRECTION ( 'NONE',  ( 0.000000000000000000, -0.000000000000000000, 1.000000000000000000 ) ) ;
#4422=ORIENTED_EDGE ( 'NONE', *, *, #3830, .F. ) ;
#4426=EDGE_CURVE ( 'NONE', #9773, #5388, #11893, .T. ) ;
#4439=ADVANCED_FACE ( 'NONE', ( #12752, #7243, #6155, #11670, #622, #5083, #3982 ), #5297, .F. ) ;
#4442=ORIENTED_EDGE ( 'NONE', *, *, #12814, .F. ) ;
#4466=LINE ( 'NONE', #12363, #7791 ) ;
#4470=EDGE_CURVE ( 'NONE', #6109, #9773, #6727, .T. ) ;
#4474=AXIS2_PLACEMENT_3D ( 'NONE', #11432, #6720, #2369 ) ;
#4476=FACE_OUTER_BOUND ( 'NONE', #3861, .T. ) ;
#4481=VECTOR ( 'NONE', #2835, 1000.000000000000000 ) ;
#4512=CARTESIAN_POINT ( 'NONE',  ( 4.999999999999999112, 8.660254037844390851, 205.0000000000000284 ) ) ;
#4520=LINE ( 'NONE', #13352, #12670 ) ;
#4523=CARTESIAN_POINT ( 'NONE',  ( 93.00000000000000000, 8.660254037844390851, 205.0000000000000284 ) ) ;
#4529=ORIENTED_EDGE ( 'NONE', *, *, #4426, .F. ) ;
#4541=EDGE_CURVE ( 'NONE', #3582, #4579, #9998, .T. ) ;
#4555=AXIS2_PLACEMENT_3D ( 'NONE', #10500, #9340, #7154 ) ;
#4560=VECTOR ( 'NONE', #9414, 1000.000000000000000 ) ;
#4568=DIRECTION ( 'NONE',  ( 0.000000000000000000, 0.000000000000000000, 1.000000000000000000 ) ) ;
#4571=AXIS2_PLACEMENT_3D ( 'NONE', #8341, #9223, #9299 ) ;
#4572=CARTESIAN_POINT ( 'NONE',  ( 259.0000000000000000, -8.660254037844389075, 205.0000000000000284 ) ) ;
#4578=ORIENTED_EDGE ( 'NONE', *, *, #2678, .F. ) ;
#4579=VERTEX_POINT ( 'NONE', #12031 ) ;
#4587=VERTEX_POINT ( 'NONE', #3262 ) ;
#4605=EDGE_CURVE ( 'NONE', #13503, #514, #2440, .T. ) ;
#4614=VERTEX_POINT ( 'NONE', #9338 ) ;
#4652=VERTEX_POINT ( 'NONE', #10344 ) ;
#4692=SURFACE_SIDE_STYLE ('',( #13594 ) ) ;
#4696=DIRECTION ( 'NONE',  ( 0.000000000000000000, 1.000000000000000000, 0.000000000000000000 ) ) ;
#4718=CARTESIAN_POINT ( 'NONE',  ( 53.33333333333330017, -20.00000000000000000, 219.8500000000001080 ) ) ;
#4735=DIRECTION ( 'NONE',  ( 0.000000000000000000, 0.000000000000000000, -1.000000000000000000 ) ) ;
#4737=LINE ( 'NONE', #1590, #13648 ) ;
#4745=DIRECTION ( 'NONE',  ( 0.000000000000000000, -1.000000000000000000, 0.000000000000000000 ) ) ;
#4748=EDGE_LOOP ( 'NONE', ( #11009, #5909 ) ) ;
#4778=DIRECTION ( 'NONE',  ( 0.000000000000000000, -0.000000000000000000, 1.000000000000000000 ) ) ;
#4796=LINE ( 'NONE', #13345, #8149 ) ;
#4809=DIRECTION ( 'NONE',  ( -0.000000000000000000, 1.000000000000000000, 0.000000000000000000 ) ) ;
#4812=VECTOR ( 'NONE', #494, 1000.000000000000000 ) ;
#4821=VERTEX_POINT ( 'NONE', #9477 ) ;
#4847=VECTOR ( 'NONE', #5742, 1000.000000000000000 ) ;
#4856=DIRECTION ( 'NONE',  ( 0.000000000000000000, -1.000000000000000000, 0.000000000000000000 ) ) ;
#4877=CARTESIAN_POINT ( 'NONE',  ( 357.0000000000000000, 8.660254037844390851, 200.0000000000000000 ) ) ;
#4879=VECTOR ( 'NONE', #10383, 1000.000000000000000 ) ;
#4884=PRODUCT_CONTEXT ( 'NONE', #4152, 'mechanical' ) ;
#4888=FACE_BOUND ( 'NONE', #925, .T. ) ;
#4899=FACE_OUTER_BOUND ( 'NONE', #9855, .T. ) ;
#4910=CARTESIAN_POINT ( 'NONE',  ( 219.9999999999999716, -15.00000000000000000, 219.8500000000001080 ) ) ;
#4919=CARTESIAN_POINT ( 'NONE',  ( 93.00000000000000000, 8.660254037844390851, 199.9990000000000236 ) ) ;
#4933=VECTOR ( 'NONE', #807, 1000.000000000000000 ) ;
#4934=AXIS2_PLACEMENT_3D ( 'NONE', #8485, #13857, #10529 ) ;
#4955=LINE ( 'NONE', #10459, #4879 ) ;
#4961=CARTESIAN_POINT ( 'NONE',  ( 219.9999999999999716, -20.00000000000000000, 219.8500000000001080 ) ) ;
#4975=EDGE_CURVE ( 'NONE', #8647, #6112, #3249, .T. ) ;
#4994=CARTESIAN_POINT ( 'NONE',  ( 170.9999999999999716, -8.660254037844389075, 199.9990000000000236 ) ) ;
#4996=CYLINDRICAL_SURFACE ( 'NONE', #1994, 2.649999999999985700 ) ;
#4998=EDGE_CURVE ( 'NONE', #514, #8720, #1107, .T. ) ;
#4999=CARTESIAN_POINT ( 'NONE',  ( 386.6666666666666288, -20.00000000000000000, 222.5000000000000853 ) ) ;
#5011=DIRECTION ( 'NONE',  ( -1.000000000000000000, -0.000000000000000000, -0.000000000000000000 ) ) ;
#5027=CARTESIAN_POINT ( 'NONE',  ( 357.0000000000000000, -8.660254037844389075, 205.0000000000000284 ) ) ;
#5036=CIRCLE ( 'NONE', #10822, 2.649999999999985700 ) ;
#5050=ORIENTED_EDGE ( 'NONE', *, *, #167, .T. ) ;
#5052=ORIENTED_EDGE ( 'NONE', *, *, #11922, .F. ) ;
#5053=VECTOR ( 'NONE', #13634, 1000.000000000000000 ) ;
#5070=CARTESIAN_POINT ( 'NONE',  ( 53.33333333333330017, -14.99999999999999822, 219.8500000000001080 ) ) ;
#5074=CARTESIAN_POINT ( 'NONE',  ( 444.9999999999999432, 8.660254037844390851, 205.0000000000000284 ) ) ;
#5077=DIRECTION ( 'NONE',  ( 1.000000000000000000, 0.000000000000000000, 0.000000000000000000 ) ) ;
#5080=DIRECTION ( 'NONE',  ( 0.000000000000000000, 1.000000000000000000, 0.000000000000000000 ) ) ;
#5083=FACE_BOUND ( 'NONE', #8608, .T. ) ;
#5086=ORIENTED_EDGE ( 'NONE', *, *, #12502, .T. ) ;
#5094=ORIENTED_EDGE ( 'NONE', *, *, #7739, .F. ) ;
#5114=AXIS2_PLACEMENT_3D ( 'NONE', #12626, #4809, #13715 ) ;
#5133=DIRECTION ( 'NONE',  ( -0.000000000000000000, 1.000000000000000000, -0.000000000000000000 ) ) ;
#5182=ORIENTED_EDGE ( 'NONE', *, *, #2089, .F. ) ;
#5197=CARTESIAN_POINT ( 'NONE',  ( 269.0000000000000000, 8.660254037844390851, 200.0000000000000000 ) ) ;
#5205=CARTESIAN_POINT ( 'NONE',  ( 219.9999999999999716, -15.00000000000000000, 225.1500000000000625 ) ) ;
#5232=ORIENTED_EDGE ( 'NONE', *, *, #12814, .T. ) ;
#5237=DIRECTION ( 'NONE',  ( 0.000000000000000000, 0.000000000000000000, -1.000000000000000000 ) ) ;
#5248=ORIENTED_EDGE ( 'NONE', *, *, #2655, .F. ) ;
#5254=LINE ( 'NONE', #2047, #2917 ) ;
#5256=DIRECTION ( 'NONE',  ( -0.000000000000000000, 1.000000000000000000, 0.000000000000000000 ) ) ;
#5273=EDGE_CURVE ( 'NONE', #3734, #6981, #3015, .T. ) ;
#5297=PLANE ( 'NONE',  #7148 ) ;
#5303=EDGE_LOOP ( 'NONE', ( #9674, #7778 ) ) ;
#5367=ORIENTED_EDGE ( 'NONE', *, *, #1576, .F. ) ;
#5375=PLANE ( 'NONE',  #5926 ) ;
#5376=VERTEX_POINT ( 'NONE', #12940 ) ;
#5388=VERTEX_POINT ( 'NONE', #7498 ) ;
#5395=EDGE_LOOP ( 'NONE', ( #5232, #11828, #7892, #2601 ) ) ;
#5400=CARTESIAN_POINT ( 'NONE',  ( 434.9999999999999432, 8.660254037844390851, 200.0000000000000000 ) ) ;
#5414=ORIENTED_EDGE ( 'NONE', *, *, #6068, .F. ) ;
#5436=ORIENTED_EDGE ( 'NONE', *, *, #1221, .F. ) ;
#5441=DIRECTION ( 'NONE',  ( 0.000000000000000000, -1.000000000000000000, 0.000000000000000000 ) ) ;
#5456=VERTEX_POINT ( 'NONE', #13014 ) ;
#5465=ORIENTED_EDGE ( 'NONE', *, *, #6767, .T. ) ;
#5466=ORIENTED_EDGE ( 'NONE', *, *, #4605, .F. ) ;
#5476=VECTOR ( 'NONE', #6072, 1000.000000000000000 ) ;
#5516=CARTESIAN_POINT ( 'NONE',  ( 170.9999999999999716, 8.660254037844390851, 199.9990000000000236 ) ) ;
#5525=EDGE_CURVE ( 'NONE', #898, #8647, #2728, .T. ) ;
#5543=VECTOR ( 'NONE', #8617, 1000.000000000000000 ) ;
#5549=CARTESIAN_POINT ( 'NONE',  ( 170.9999999999999716, -8.660254037844389075, 200.0000000000000000 ) ) ;
#5554=DIRECTION ( 'NONE',  ( -0.000000000000000000, 0.000000000000000000, 1.000000000000000000 ) ) ;
#5555=CARTESIAN_POINT ( 'NONE',  ( 82.99999999999998579, -8.660254037844389075, 199.9990000000000236 ) ) ;
#5559=CARTESIAN_POINT ( 'NONE',  ( 82.99999999999998579, -8.660254037844389075, 205.0000000000000284 ) ) ;
#5571=AXIS2_PLACEMENT_3D ( 'NONE', #6812, #2607, #5793 ) ;
#5576=CARTESIAN_POINT ( 'NONE',  ( 470.0000000000000000, 0.000000000000000000, 205.0000000000000284 ) ) ;
#5580=EDGE_LOOP ( 'NONE', ( #7604, #13788, #11944, #8459 ) ) ;
#5592=ORIENTED_EDGE ( 'NONE', *, *, #11142, .F. ) ;
#5594=CARTESIAN_POINT ( 'NONE',  ( 219.9999999999999716, -15.00000000000000000, 222.5000000000000853 ) ) ;
#5600=ORIENTED_EDGE ( 'NONE', *, *, #10191, .T. ) ;
#5621=ORIENTED_EDGE ( 'NONE', *, *, #2163, .T. ) ;
#5624=DIRECTION ( 'NONE',  ( 0.000000000000000000, 0.000000000000000000, 1.000000000000000000 ) ) ;
#5643=VERTEX_POINT ( 'NONE', #8944 ) ;
#5665=CARTESIAN_POINT ( 'NONE',  ( 269.0000000000000000, 8.660254037844390851, 200.0000000000000000 ) ) ;
#5679=VERTEX_POINT ( 'NONE', #5027 ) ;
#5680=CARTESIAN_POINT ( 'NONE',  ( 170.9999999999999716, 8.660254037844390851, 200.0000000000000000 ) ) ;
#5685=EDGE_CURVE ( 'NONE', #806, #611, #8348, .T. ) ;
#5686=CARTESIAN_POINT ( 'NONE',  ( 259.0000000000000000, -8.660254037844389075, 200.0000000000000000 ) ) ;
#5702=VECTOR ( 'NONE', #6273, 1000.000000000000000 ) ;
#5711=PLANE ( 'NONE',  #8585 ) ;
#5717=VECTOR ( 'NONE', #11420, 1000.000000000000000 ) ;
#5724=FACE_OUTER_BOUND ( 'NONE', #8421, .T. ) ;
#5742=DIRECTION ( 'NONE',  ( -0.000000000000000000, -0.000000000000000000, -1.000000000000000000 ) ) ;
#5744=DIRECTION ( 'NONE',  ( -0.000000000000000000, 1.000000000000000000, -0.000000000000000000 ) ) ;
#5772=ORIENTED_EDGE ( 'NONE', *, *, #340, .T. ) ;
#5788=ORIENTED_EDGE ( 'NONE', *, *, #12301, .F. ) ;
#5790=LINE ( 'NONE', #13614, #8001 ) ;
#5793=DIRECTION ( 'NONE',  ( 0.000000000000000000, 0.000000000000000000, 1.000000000000000000 ) ) ;
#5804=LINE ( 'NONE', #10085, #11941 ) ;
#5823=VERTEX_POINT ( 'NONE', #2916 ) ;
#5852=DIRECTION ( 'NONE',  ( -1.000000000000000000, 0.000000000000000000, -0.000000000000000000 ) ) ;
#5858=CARTESIAN_POINT ( 'NONE',  ( 303.3333333333333144, -15.00000000000000000, 219.8500000000001080 ) ) ;
#5861=ORIENTED_EDGE ( 'NONE', *, *, #5273, .T. ) ;
#5862=DIRECTION ( 'NONE',  ( -0.000000000000000000, -0.000000000000000000, 1.000000000000000000 ) ) ;
#5864=LINE ( 'NONE', #1715, #7817 ) ;
#5886=LINE ( 'NONE', #10037, #2952 ) ;
#5893=ORIENTED_EDGE ( 'NONE', *, *, #4470, .F. ) ;
#5909=ORIENTED_EDGE ( 'NONE', *, *, #308, .F. ) ;
#5910=( NAMED_UNIT ( * ) SI_UNIT ( $, .STERADIAN. ) SOLID_ANGLE_UNIT ( ) );
#5915=ORIENTED_EDGE ( 'NONE', *, *, #11473, .F. ) ;
#5926=AXIS2_PLACEMENT_3D ( 'NONE', #1952, #10964, #10677 ) ;
#5931=LINE ( 'NONE', #7883, #1521 ) ;
#5954=CARTESIAN_POINT ( 'NONE',  ( 269.0000000000000000, 8.660254037844390851, 199.9990000000000236 ) ) ;
#5963=ADVANCED_FACE ( 'NONE', ( #7828 ), #13751, .F. ) ;
#5971=CARTESIAN_POINT ( 'NONE',  ( 347.0000000000000000, 8.660254037844390851, 205.0000000000000284 ) ) ;
#5981=PLANE ( 'NONE',  #8370 ) ;
#5996=AXIS2_PLACEMENT_3D ( 'NONE', #3788, #335, #11259 ) ;
#6004=DIRECTION ( 'NONE',  ( 0.000000000000000000, 0.000000000000000000, 1.000000000000000000 ) ) ;
#6006=CARTESIAN_POINT ( 'NONE',  ( 269.0000000000000000, -8.660254037844389075, 199.9990000000000236 ) ) ;
#6017=ORIENTED_EDGE ( 'NONE', *, *, #1221, .T. ) ;
#6032=EDGE_CURVE ( 'NONE', #486, #2517, #12594, .T. ) ;
#6035=ADVANCED_FACE ( 'NONE', ( #3681 ), #8091, .F. ) ;
#6041=ORIENTED_EDGE ( 'NONE', *, *, #11728, .F. ) ;
#6048=EDGE_CURVE ( 'NONE', #8647, #898, #1757, .T. ) ;
#6053=ADVANCED_FACE ( 'NONE', ( #303 ), #9407, .F. ) ;
#6056=ORIENTED_EDGE ( 'NONE', *, *, #6068, .T. ) ;
#6060=DIRECTION ( 'NONE',  ( -0.000000000000000000, -0.000000000000000000, 1.000000000000000000 ) ) ;
#6068=EDGE_CURVE ( 'NONE', #7334, #7167, #8231, .T. ) ;
#6072=DIRECTION ( 'NONE',  ( -0.000000000000000000, -0.000000000000000000, 1.000000000000000000 ) ) ;
#6074=DIRECTION ( 'NONE',  ( -0.000000000000000000, 1.000000000000000000, -0.000000000000000000 ) ) ;
#6090=EDGE_LOOP ( 'NONE', ( #696, #8694, #10235, #8014 ) ) ;
#6091=CARTESIAN_POINT ( 'NONE',  ( 181.0000000000000000, 8.660254037844390851, 199.9990000000000236 ) ) ;
#6109=VERTEX_POINT ( 'NONE', #2812 ) ;
#6112=VERTEX_POINT ( 'NONE', #5070 ) ;
#6119=EDGE_CURVE ( 'NONE', #13937, #2529, #10570, .T. ) ;
#6145=ORIENTED_EDGE ( 'NONE', *, *, #2511, .F. ) ;
#6151=DIRECTION ( 'NONE',  ( 1.000000000000000000, 0.000000000000000000, 0.000000000000000000 ) ) ;
#6155=FACE_OUTER_BOUND ( 'NONE', #11082, .T. ) ;
#6158=ORIENTED_EDGE ( 'NONE', *, *, #14212, .F. ) ;
#6164=EDGE_LOOP ( 'NONE', ( #2961, #3431 ) ) ;
#6166=ORIENTED_EDGE ( 'NONE', *, *, #3754, .F. ) ;
#6169=ORIENTED_EDGE ( 'NONE', *, *, #1553, .T. ) ;
#6172=EDGE_CURVE ( 'NONE', #8606, #6112, #3405, .T. ) ;
#6173=FACE_OUTER_BOUND ( 'NONE', #8420, .T. ) ;
#6177=EDGE_LOOP ( 'NONE', ( #9451, #9774, #261, #6911 ) ) ;
#6179=ORIENTED_EDGE ( 'NONE', *, *, #1576, .T. ) ;
#6186=ORIENTED_EDGE ( 'NONE', *, *, #6640, .T. ) ;
#6194=LINE ( 'NONE', #12053, #6761 ) ;
#6200=AXIS2_PLACEMENT_3D ( 'NONE', #11902, #12766, #554 ) ;
#6202=AXIS2_PLACEMENT_3D ( 'NONE', #6673, #3208, #4568 ) ;
#6217=CARTESIAN_POINT ( 'NONE',  ( 136.6666666666666288, -14.99999999999999822, 222.5000000000000853 ) ) ;
#6220=ORIENTED_EDGE ( 'NONE', *, *, #11262, .F. ) ;
#6234=DIRECTION ( 'NONE',  ( 1.000000000000000000, 0.000000000000000000, 0.000000000000000000 ) ) ;
#6236=LINE ( 'NONE', #143, #4254 ) ;
#6259=ORIENTED_EDGE ( 'NONE', *, *, #3043, .F. ) ;
#6269=ORIENTED_EDGE ( 'NONE', *, *, #13228, .T. ) ;
#6273=DIRECTION ( 'NONE',  ( -0.000000000000000000, 1.000000000000000000, -0.000000000000000000 ) ) ;
#6303=DIRECTION ( 'NONE',  ( 0.000000000000000000, 0.000000000000000000, -1.000000000000000000 ) ) ;
#6306=VECTOR ( 'NONE', #7417, 1000.000000000000000 ) ;
#6309=VERTEX_POINT ( 'NONE', #8246 ) ;
#6311=ORIENTED_EDGE ( 'NONE', *, *, #12885, .F. ) ;
#6315=CARTESIAN_POINT ( 'NONE',  ( 93.00000000000000000, -8.660254037844389075, 205.0000000000000284 ) ) ;
#6319=CARTESIAN_POINT ( 'NONE',  ( 357.0000000000000000, 8.660254037844390851, 199.9990000000000236 ) ) ;
#6320=PRODUCT_DEFINITION_FORMATION_WITH_SPECIFIED_SOURCE ( 'ANY', '', #4382, .NOT_KNOWN. ) ;
#6331=EDGE_CURVE ( 'NONE', #2838, #3406, #8032, .T. ) ;
#6332=DIRECTION ( 'NONE',  ( -0.000000000000000000, 0.000000000000000000, 1.000000000000000000 ) ) ;
#6343=EDGE_CURVE ( 'NONE', #6309, #8482, #12471, .T. ) ;
#6351=CARTESIAN_POINT ( 'NONE',  ( 82.99999999999998579, 8.660254037844390851, 205.0000000000000284 ) ) ;
#6355=ORIENTED_EDGE ( 'NONE', *, *, #12301, .T. ) ;
#6357=EDGE_CURVE ( 'NONE', #930, #3366, #7956, .T. ) ;
#6385=CARTESIAN_POINT ( 'NONE',  ( 347.0000000000000000, 8.660254037844390851, 200.0000000000000000 ) ) ;
#6396=ORIENTED_EDGE ( 'NONE', *, *, #2963, .F. ) ;
#6409=LINE ( 'NONE', #4163, #359 ) ;
#6412=VECTOR ( 'NONE', #11939, 1000.000000000000000 ) ;
#6416=ORIENTED_EDGE ( 'NONE', *, *, #12946, .T. ) ;
#6420=VECTOR ( 'NONE', #3797, 1000.000000000000000 ) ;
#6469=ORIENTED_EDGE ( 'NONE', *, *, #1797, .T. ) ;
#6475=ORIENTED_EDGE ( 'NONE', *, *, #6343, .F. ) ;
#6484=EDGE_CURVE ( 'NONE', #7334, #11965, #10347, .T. ) ;
#6492=CARTESIAN_POINT ( 'NONE',  ( 386.6666666666666288, -15.00000000000000000, 225.1500000000000625 ) ) ;
#6497=VERTEX_POINT ( 'NONE', #13510 ) ;
#6499=ADVANCED_FACE ( 'NONE', ( #2283 ), #12292, .F. ) ;
#6505=VECTOR ( 'NONE', #7081, 1000.000000000000000 ) ;
#6516=ADVANCED_FACE ( 'NONE', ( #2498 ), #10048, .F. ) ;
#6521=EDGE_LOOP ( 'NONE', ( #12767, #12332 ) ) ;
#6537=AXIS2_PLACEMENT_3D ( 'NONE', #3280, #9946, #12861 ) ;
#6549=ORIENTED_EDGE ( 'NONE', *, *, #6048, .F. ) ;
#6557=DIRECTION ( 'NONE',  ( 0.000000000000000000, 0.000000000000000000, 1.000000000000000000 ) ) ;
#6558=EDGE_CURVE ( 'NONE', #6497, #6109, #10257, .T. ) ;
#6562=ORIENTED_EDGE ( 'NONE', *, *, #8747, .T. ) ;
#6565=EDGE_CURVE ( 'NONE', #7514, #3844, #13577, .T. ) ;
#6568=VERTEX_POINT ( 'NONE', #1534 ) ;
#6585=FACE_OUTER_BOUND ( 'NONE', #10430, .T. ) ;
#6608=ORIENTED_EDGE ( 'NONE', *, *, #5273, .F. ) ;
#6610=DIRECTION ( 'NONE',  ( -0.000000000000000000, 1.000000000000000000, -0.000000000000000000 ) ) ;
#6617=ORIENTED_EDGE ( 'NONE', *, *, #10733, .T. ) ;
#6622=AXIS2_PLACEMENT_3D ( 'NONE', #6694, #13288, #8938 ) ;
#6628=ORIENTED_EDGE ( 'NONE', *, *, #6989, .F. ) ;
#6629=CARTESIAN_POINT ( 'NONE',  ( 4.999999999999999112, 8.660254037844390851, 200.0000000000000000 ) ) ;
#6640=EDGE_CURVE ( 'NONE', #611, #6568, #1606, .T. ) ;
#6651=FACE_BOUND ( 'NONE', #4748, .T. ) ;
#6663=CARTESIAN_POINT ( 'NONE',  ( 4.999999999999999112, 8.660254037844390851, 200.0000000000000000 ) ) ;
#6673=CARTESIAN_POINT ( 'NONE',  ( 136.6666666666666288, -20.00000000000000000, 222.5000000000000853 ) ) ;
#6681=CYLINDRICAL_SURFACE ( 'NONE', #876, 2.649999999999985700 ) ;
#6682=DIRECTION ( 'NONE',  ( -0.000000000000000000, 0.000000000000000000, 1.000000000000000000 ) ) ;
#6694=CARTESIAN_POINT ( 'NONE',  ( 386.6666666666666288, -14.99999999999999822, 222.5000000000000853 ) ) ;
#6703=AXIS2_PLACEMENT_3D ( 'NONE', #9357, #2538, #393 ) ;
#6720=DIRECTION ( 'NONE',  ( -0.000000000000000000, 1.000000000000000000, -0.000000000000000000 ) ) ;
#6727=LINE ( 'NONE', #3191, #12492 ) ;
#6748=CARTESIAN_POINT ( 'NONE',  ( 53.33333333333330017, -20.00000000000000000, 222.5000000000000853 ) ) ;
#6753=LINE ( 'NONE', #1366, #3089 ) ;
#6759=DIRECTION ( 'NONE',  ( 0.000000000000000000, 0.000000000000000000, 1.000000000000000000 ) ) ;
#6761=VECTOR ( 'NONE', #2868, 1000.000000000000000 ) ;
#6767=EDGE_CURVE ( 'NONE', #13397, #10177, #5254, .T. ) ;
#6774=EDGE_LOOP ( 'NONE', ( #6562, #7917, #13841, #13032 ) ) ;
#6778=ORIENTED_EDGE ( 'NONE', *, *, #7739, .T. ) ;
#6780=VECTOR ( 'NONE', #12337, 1000.000000000000000 ) ;
#6795=LINE ( 'NONE', #2435, #1661 ) ;
#6798=EDGE_LOOP ( 'NONE', ( #14133, #3611, #6259, #8385 ) ) ;
#6807=ORIENTED_EDGE ( 'NONE', *, *, #3485, .F. ) ;
#6812=CARTESIAN_POINT ( 'NONE',  ( 136.6666666666666288, -15.00000000000000000, 222.5000000000000853 ) ) ;
#6819=DIRECTION ( 'NONE',  ( 0.000000000000000000, 0.000000000000000000, 1.000000000000000000 ) ) ;
#6830=( LENGTH_UNIT ( ) NAMED_UNIT ( * ) SI_UNIT ( .MILLI., .METRE. ) );
#6842=CARTESIAN_POINT ( 'NONE',  ( 434.9999999999999432, -8.660254037844389075, 199.9990000000000236 ) ) ;
#6853=ORIENTED_EDGE ( 'NONE', *, *, #2637, .T. ) ;
#6856=DIRECTION ( 'NONE',  ( 0.000000000000000000, 1.000000000000000000, 0.000000000000000000 ) ) ;
#6875=PLANE ( 'NONE',  #7313 ) ;
#6888=ORIENTED_EDGE ( 'NONE', *, *, #4353, .T. ) ;
#6903=DIRECTION ( 'NONE',  ( -0.000000000000000000, 1.000000000000000000, -0.000000000000000000 ) ) ;
#6911=ORIENTED_EDGE ( 'NONE', *, *, #7618, .T. ) ;
#6967=ORIENTED_EDGE ( 'NONE', *, *, #11890, .F. ) ;
#6981=VERTEX_POINT ( 'NONE', #3635 ) ;
#6982=LINE ( 'NONE', #5559, #10672 ) ;
#6989=EDGE_CURVE ( 'NONE', #12864, #4316, #808, .T. ) ;
#7002=( NAMED_UNIT ( * ) PLANE_ANGLE_UNIT ( ) SI_UNIT ( $, .RADIAN. ) );
#7004=FACE_OUTER_BOUND ( 'NONE', #4237, .T. ) ;
#7016=ADVANCED_FACE ( 'NONE', ( #12200 ), #12276, .F. ) ;
#7018=DIRECTION ( 'NONE',  ( 0.000000000000000000, 0.000000000000000000, 1.000000000000000000 ) ) ;
#7034=VERTEX_POINT ( 'NONE', #1732 ) ;
#7055=ORIENTED_EDGE ( 'NONE', *, *, #12154, .T. ) ;
#7073=EDGE_CURVE ( 'NONE', #13284, #10673, #7179, .T. ) ;
#7081=DIRECTION ( 'NONE',  ( -0.000000000000000000, 1.000000000000000000, -0.000000000000000000 ) ) ;
#7104=CARTESIAN_POINT ( 'NONE',  ( 347.0000000000000000, -8.660254037844389075, 200.0000000000000000 ) ) ;
#7113=VERTEX_POINT ( 'NONE', #9511 ) ;
#7123=ORIENTED_EDGE ( 'NONE', *, *, #6172, .T. ) ;
#7142=ORIENTED_EDGE ( 'NONE', *, *, #4470, .T. ) ;
#7148=AXIS2_PLACEMENT_3D ( 'NONE', #8396, #9718, #12827 ) ;
#7153=DIRECTION ( 'NONE',  ( -0.000000000000000000, -0.000000000000000000, 1.000000000000000000 ) ) ;
#7154=DIRECTION ( 'NONE',  ( 0.000000000000000000, -0.000000000000000000, -1.000000000000000000 ) ) ;
#7157=DIRECTION ( 'NONE',  ( -0.000000000000000000, 1.000000000000000000, -0.000000000000000000 ) ) ;
#7163=LINE ( 'NONE', #11594, #11175 ) ;
#7164=DIRECTION ( 'NONE',  ( -1.000000000000000000, 0.000000000000000000, 0.000000000000000000 ) ) ;
#7167=VERTEX_POINT ( 'NONE', #1659 ) ;
#7171=VERTEX_POINT ( 'NONE', #10816 ) ;
#7179=LINE ( 'NONE', #7256, #9635 ) ;
#7180=PLANE ( 'NONE',  #3881 ) ;
#7184=CARTESIAN_POINT ( 'NONE',  ( 4.999999999999999112, 8.660254037844390851, 199.9990000000000236 ) ) ;
#7191=ADVANCED_FACE ( 'NONE', ( #13058 ), #703, .F. ) ;
#7192=ORIENTED_EDGE ( 'NONE', *, *, #6558, .F. ) ;
#7197=ORIENTED_EDGE ( 'NONE', *, *, #6331, .F. ) ;
#7203=ADVANCED_FACE ( 'NONE', ( #913 ), #5375, .F. ) ;
#7210=CARTESIAN_POINT ( 'NONE',  ( 0.000000000000000000, -15.00000000000000000, 205.0000000000000284 ) ) ;
#7211=ORIENTED_EDGE ( 'NONE', *, *, #11839, .T. ) ;
#7216=DIRECTION ( 'NONE',  ( -0.000000000000000000, 1.000000000000000000, -0.000000000000000000 ) ) ;
#7227=AXIS2_PLACEMENT_3D ( 'NONE', #3153, #2040, #2188 ) ;
#7243=FACE_BOUND ( 'NONE', #12129, .T. ) ;
#7256=CARTESIAN_POINT ( 'NONE',  ( 170.9999999999999716, -8.660254037844389075, 200.0000000000000000 ) ) ;
#7268=VERTEX_POINT ( 'NONE', #12990 ) ;
#7289=CARTESIAN_POINT ( 'NONE',  ( 219.9999999999999716, -14.99999999999999822, 222.5000000000000853 ) ) ;
#7297=CIRCLE ( 'NONE', #788, 2.649999999999985700 ) ;
#7308=DIRECTION ( 'NONE',  ( 0.000000000000000000, 0.000000000000000000, 1.000000000000000000 ) ) ;
#7309=LINE ( 'NONE', #3910, #10871 ) ;
#7313=AXIS2_PLACEMENT_3D ( 'NONE', #10215, #1277, #3415 ) ;
#7318=VECTOR ( 'NONE', #12602, 1000.000000000000000 ) ;
#7331=VECTOR ( 'NONE', #8442, 1000.000000000000000 ) ;
#7334=VERTEX_POINT ( 'NONE', #13269 ) ;
#7350=LINE ( 'NONE', #8433, #3729 ) ;
#7362=CARTESIAN_POINT ( 'NONE',  ( 357.0000000000000000, -8.660254037844389075, 199.9990000000000236 ) ) ;
#7381=ADVANCED_FACE ( 'NONE', ( #2240 ), #6875, .F. ) ;
#7397=LINE ( 'NONE', #6385, #3879 ) ;
#7413=FACE_BOUND ( 'NONE', #638, .T. ) ;
#7417=DIRECTION ( 'NONE',  ( -0.000000000000000000, 1.000000000000000000, -0.000000000000000000 ) ) ;
#7423=ORIENTED_EDGE ( 'NONE', *, *, #13053, .F. ) ;
#7461=DIRECTION ( 'NONE',  ( 1.000000000000000000, 0.000000000000000000, 0.000000000000000000 ) ) ;
#7474=CARTESIAN_POINT ( 'NONE',  ( 259.0000000000000000, -8.660254037844389075, 199.9990000000000236 ) ) ;
#7498=CARTESIAN_POINT ( 'NONE',  ( 269.0000000000000000, -8.660254037844389075, 205.0000000000000284 ) ) ;
#7499=ORIENTED_EDGE ( 'NONE', *, *, #10908, .T. ) ;
#7500=ADVANCED_FACE ( 'NONE', ( #9197 ), #4996, .F. ) ;
#7514=VERTEX_POINT ( 'NONE', #10578 ) ;
#7545=ORIENTED_EDGE ( 'NONE', *, *, #4605, .T. ) ;
#7551=ORIENTED_EDGE ( 'NONE', *, *, #7790, .F. ) ;
#7562=EDGE_CURVE ( 'NONE', #1151, #4587, #12672, .T. ) ;
#7570=EDGE_CURVE ( 'NONE', #4821, #7268, #8319, .T. ) ;
#7591=VECTOR ( 'NONE', #10455, 1000.000000000000000 ) ;
#7592=CARTESIAN_POINT ( 'NONE',  ( -5.000000000000000888, 8.660254037844390851, 200.0000000000000000 ) ) ;
#7603=ADVANCED_FACE ( 'NONE', ( #10283 ), #13757, .F. ) ;
#7604=ORIENTED_EDGE ( 'NONE', *, *, #4375, .F. ) ;
#7612=DIRECTION ( 'NONE',  ( -0.000000000000000000, 1.000000000000000000, -0.000000000000000000 ) ) ;
#7618=EDGE_CURVE ( 'NONE', #2842, #10535, #5036, .T. ) ;
#7631=DIRECTION ( 'NONE',  ( -0.000000000000000000, 1.000000000000000000, -0.000000000000000000 ) ) ;
#7643=ORIENTED_EDGE ( 'NONE', *, *, #7790, .T. ) ;
#7649=VECTOR ( 'NONE', #9529, 1000.000000000000000 ) ;
#7657=ORIENTED_EDGE ( 'NONE', *, *, #10621, .T. ) ;
#7661=ORIENTED_EDGE ( 'NONE', *, *, #1553, .F. ) ;
#7670=VECTOR ( 'NONE', #11723, 1000.000000000000000 ) ;
#7676=ORIENTED_EDGE ( 'NONE', *, *, #6558, .T. ) ;
#7679=CARTESIAN_POINT ( 'NONE',  ( -5.000000000000000888, 8.660254037844390851, 200.0000000000000000 ) ) ;
#7694=ORIENTED_EDGE ( 'NONE', *, *, #12414, .T. ) ;
#7697=CARTESIAN_POINT ( 'NONE',  ( 347.0000000000000000, -8.660254037844389075, 199.9990000000000236 ) ) ;
#7724=PRODUCT_DEFINITION_SHAPE ( 'NONE', 'NONE',  #13657 ) ;
#7733=CARTESIAN_POINT ( 'NONE',  ( 4.999999999999999112, -8.660254037844389075, 199.9990000000000236 ) ) ;
#7739=EDGE_CURVE ( 'NONE', #13503, #2327, #10800, .T. ) ;
#7778=ORIENTED_EDGE ( 'NONE', *, *, #6048, .T. ) ;
#7790=EDGE_CURVE ( 'NONE', #4316, #12864, #2476, .T. ) ;
#7791=VECTOR ( 'NONE', #8887, 1000.000000000000000 ) ;
#7817=VECTOR ( 'NONE', #6151, 1000.000000000000000 ) ;
#7828=FACE_OUTER_BOUND ( 'NONE', #8060, .T. ) ;
#7832=CARTESIAN_POINT ( 'NONE',  ( 219.9999999999999716, -14.99999999999999822, 222.5000000000000853 ) ) ;
#7837=EDGE_LOOP ( 'NONE', ( #13485, #6311 ) ) ;
#7851=EDGE_LOOP ( 'NONE', ( #3675, #7676, #9514, #14293 ) ) ;
#7857=VECTOR ( 'NONE', #10791, 1000.000000000000000 ) ;
#7858=CARTESIAN_POINT ( 'NONE',  ( 434.9999999999999432, 8.660254037844390851, 200.0000000000000000 ) ) ;
#7863=AXIS2_PLACEMENT_3D ( 'NONE', #4137, #9725, #8554 ) ;
#7883=CARTESIAN_POINT ( 'NONE',  ( 259.0000000000000000, 8.660254037844390851, 200.0000000000000000 ) ) ;
#7886=DIRECTION ( 'NONE',  ( -0.000000000000000000, -0.000000000000000000, 1.000000000000000000 ) ) ;
#7892=ORIENTED_EDGE ( 'NONE', *, *, #4353, .F. ) ;
#7908=DIRECTION ( 'NONE',  ( 0.000000000000000000, 0.000000000000000000, 1.000000000000000000 ) ) ;
#7917=ORIENTED_EDGE ( 'NONE', *, *, #1350, .T. ) ;
#7921=EDGE_LOOP ( 'NONE', ( #8051, #1698 ) ) ;
#7923=DIRECTION ( 'NONE',  ( -0.000000000000000000, 1.000000000000000000, -0.000000000000000000 ) ) ;
#7926=AXIS2_PLACEMENT_3D ( 'NONE', #6319, #1957, #5237 ) ;
#7928=CARTESIAN_POINT ( 'NONE',  ( -5.000000000000000888, 8.660254037844390851, 199.9990000000000236 ) ) ;
#7952=DIRECTION ( 'NONE',  ( -0.000000000000000000, -0.000000000000000000, 1.000000000000000000 ) ) ;
#7956=LINE ( 'NONE', #10224, #2950 ) ;
#7979=VECTOR ( 'NONE', #13447, 1000.000000000000000 ) ;
#7987=DIRECTION ( 'NONE',  ( 0.000000000000000000, -1.000000000000000000, 0.000000000000000000 ) ) ;
#8000=( LENGTH_UNIT ( ) NAMED_UNIT ( * ) SI_UNIT ( .MILLI., .METRE. ) );
#8001=VECTOR ( 'NONE', #7952, 1000.000000000000000 ) ;
#8005=AXIS2_PLACEMENT_3D ( 'NONE', #12264, #5852, #2739 ) ;
#8013=VECTOR ( 'NONE', #12607, 1000.000000000000000 ) ;
#8014=ORIENTED_EDGE ( 'NONE', *, *, #10729, .F. ) ;
#8032=LINE ( 'NONE', #13618, #14278 ) ;
#8038=VERTEX_POINT ( 'NONE', #8874 ) ;
#8043=EDGE_LOOP ( 'NONE', ( #5893, #7192, #13242, #4529 ) ) ;
#8051=ORIENTED_EDGE ( 'NONE', *, *, #10592, .T. ) ;
#8060=EDGE_LOOP ( 'NONE', ( #6778, #7657, #11410, #5466 ) ) ;
#8063=DIRECTION ( 'NONE',  ( 0.000000000000000000, 0.000000000000000000, 1.000000000000000000 ) ) ;
#8066=EDGE_LOOP ( 'NONE', ( #5621, #7211, #12066, #8773 ) ) ;
#8070=EDGE_CURVE ( 'NONE', #3366, #4821, #2127, .T. ) ;
#8072=CARTESIAN_POINT ( 'NONE',  ( 434.9999999999999432, 8.660254037844390851, 205.0000000000000284 ) ) ;
#8083=CARTESIAN_POINT ( 'NONE',  ( 357.0000000000000000, -8.660254037844389075, 200.0000000000000000 ) ) ;
#8091=PLANE ( 'NONE',  #4555 ) ;
#8141=DIRECTION ( 'NONE',  ( 0.000000000000000000, 0.000000000000000000, 1.000000000000000000 ) ) ;
#8149=VECTOR ( 'NONE', #194, 1000.000000000000000 ) ;
#8154=VECTOR ( 'NONE', #12806, 1000.000000000000000 ) ;
#8167=EDGE_CURVE ( 'NONE', #5643, #6568, #6409, .T. ) ;
#8172=CARTESIAN_POINT ( 'NONE',  ( 170.9999999999999716, 8.660254037844390851, 205.0000000000000284 ) ) ;
#8173=CARTESIAN_POINT ( 'NONE',  ( 82.99999999999998579, -8.660254037844389075, 205.0000000000000284 ) ) ;
#8180=ORIENTED_EDGE ( 'NONE', *, *, #8367, .T. ) ;
#8185=PLANE ( 'NONE',  #11202 ) ;
#8203=CARTESIAN_POINT ( 'NONE',  ( -30.00000000000002842, 15.00000000000000000, 200.0000000000000000 ) ) ;
#8231=LINE ( 'NONE', #11581, #12194 ) ;
#8246=CARTESIAN_POINT ( 'NONE',  ( 347.0000000000000000, 8.660254037844390851, 200.0000000000000000 ) ) ;
#8254=DIRECTION ( 'NONE',  ( 0.000000000000000000, 0.000000000000000000, -1.000000000000000000 ) ) ;
#8256=DIRECTION ( 'NONE',  ( -0.000000000000000000, -0.000000000000000000, 1.000000000000000000 ) ) ;
#8260=VECTOR ( 'NONE', #11558, 1000.000000000000000 ) ;
#8265=EDGE_CURVE ( 'NONE', #12687, #8456, #5886, .T. ) ;
#8275=CARTESIAN_POINT ( 'NONE',  ( -5.000000000000000888, -8.660254037844389075, 205.0000000000000284 ) ) ;
#8289=DIRECTION ( 'NONE',  ( 0.000000000000000000, -1.000000000000000000, 0.000000000000000000 ) ) ;
#8291=LINE ( 'NONE', #8072, #2587 ) ;
#8318=ORIENTED_EDGE ( 'NONE', *, *, #1250, .T. ) ;
#8319=LINE ( 'NONE', #1426, #13573 ) ;
#8336=CARTESIAN_POINT ( 'NONE',  ( 347.0000000000000000, 8.660254037844390851, 205.0000000000000284 ) ) ;
#8341=CARTESIAN_POINT ( 'NONE',  ( 0.000000000000000000, -20.00000000000000000, 0.000000000000000000 ) ) ;
#8347=ADVANCED_FACE ( 'NONE', ( #487, #12773, #559, #3929, #9444, #12560 ), #13710, .F. ) ;
#8348=LINE ( 'NONE', #7184, #4812 ) ;
#8350=EDGE_LOOP ( 'NONE', ( #1544, #5772, #3413, #396 ) ) ;
#8361=DIRECTION ( 'NONE',  ( 0.000000000000000000, -0.000000000000000000, 1.000000000000000000 ) ) ;
#8367=EDGE_CURVE ( 'NONE', #8038, #3734, #2695, .T. ) ;
#8370=AXIS2_PLACEMENT_3D ( 'NONE', #10477, #9166, #10402 ) ;
#8385=ORIENTED_EDGE ( 'NONE', *, *, #12946, .F. ) ;
#8396=CARTESIAN_POINT ( 'NONE',  ( 0.000000000000000000, 0.000000000000000000, 205.0000000000000284 ) ) ;
#8420=EDGE_LOOP ( 'NONE', ( #12418, #1533, #1228, #3181 ) ) ;
#8421=EDGE_LOOP ( 'NONE', ( #13868, #10246, #744, #7123 ) ) ;
#8425=ORIENTED_EDGE ( 'NONE', *, *, #7073, .F. ) ;
#8433=CARTESIAN_POINT ( 'NONE',  ( -5.000000000000000888, -8.660254037844389075, 200.0000000000000000 ) ) ;
#8438=ORIENTED_EDGE ( 'NONE', *, *, #10705, .T. ) ;
#8442=DIRECTION ( 'NONE',  ( 1.000000000000000000, 0.000000000000000000, 0.000000000000000000 ) ) ;
#8446=DIRECTION ( 'NONE',  ( -0.000000000000000000, -0.000000000000000000, 1.000000000000000000 ) ) ;
#8456=VERTEX_POINT ( 'NONE', #10892 ) ;
#8459=ORIENTED_EDGE ( 'NONE', *, *, #1321, .F. ) ;
#8482=VERTEX_POINT ( 'NONE', #3210 ) ;
#8485=CARTESIAN_POINT ( 'NONE',  ( 4.999999999999999112, 8.660254037844390851, 199.9990000000000236 ) ) ;
#8507=UNCERTAINTY_MEASURE_WITH_UNIT (LENGTH_MEASURE( 1.000000000000000082E-05 ), #6830, 'distance_accuracy_value', 'NONE');
#8531=CARTESIAN_POINT ( 'NONE',  ( -30.00000000000002842, -15.00000000000000000, 200.0000000000000000 ) ) ;
#8540=LINE ( 'NONE', #7592, #11375 ) ;
#8548=AXIS2_PLACEMENT_3D ( 'NONE', #10664, #9497, #545 ) ;
#8554=DIRECTION ( 'NONE',  ( -0.000000000000000000, 0.000000000000000000, 1.000000000000000000 ) ) ;
#8558=VECTOR ( 'NONE', #9261, 1000.000000000000000 ) ;
#8565=VECTOR ( 'NONE', #7153, 1000.000000000000000 ) ;
#8585=AXIS2_PLACEMENT_3D ( 'NONE', #4994, #2816, #1712 ) ;
#8606=VERTEX_POINT ( 'NONE', #2532 ) ;
#8608=EDGE_LOOP ( 'NONE', ( #13112, #13612, #10066, #2999 ) ) ;
#8613=CARTESIAN_POINT ( 'NONE',  ( 303.3333333333333144, -14.99999999999999822, 222.5000000000000853 ) ) ;
#8614=ADVANCED_FACE ( 'NONE', ( #1356 ), #13473, .F. ) ;
#8617=DIRECTION ( 'NONE',  ( -0.000000000000000000, -0.000000000000000000, 1.000000000000000000 ) ) ;
#8647=VERTEX_POINT ( 'NONE', #4718 ) ;
#8651=ORIENTED_EDGE ( 'NONE', *, *, #167, .F. ) ;
#8654=ORIENTED_EDGE ( 'NONE', *, *, #11473, .T. ) ;
#8663=VERTEX_POINT ( 'NONE', #11447 ) ;
#8694=ORIENTED_EDGE ( 'NONE', *, *, #4375, .T. ) ;
#8702=EDGE_CURVE ( 'NONE', #7268, #5823, #5864, .T. ) ;
#8707=FACE_OUTER_BOUND ( 'NONE', #8797, .T. ) ;
#8717=ORIENTED_EDGE ( 'NONE', *, *, #7570, .F. ) ;
#8720=VERTEX_POINT ( 'NONE', #8173 ) ;
#8747=EDGE_CURVE ( 'NONE', #7034, #5388, #3829, .T. ) ;
#8772=FACE_OUTER_BOUND ( 'NONE', #10904, .T. ) ;
#8773=ORIENTED_EDGE ( 'NONE', *, *, #13158, .F. ) ;
#8782=CARTESIAN_POINT ( 'NONE',  ( 53.33333333333330017, -14.99999999999999822, 222.5000000000000853 ) ) ;
#8786=VERTEX_POINT ( 'NONE', #9785 ) ;
#8789=CYLINDRICAL_SURFACE ( 'NONE', #544, 2.649999999999985700 ) ;
#8797=EDGE_LOOP ( 'NONE', ( #11844, #3335, #6617, #7643 ) ) ;
#8801=ADVANCED_FACE ( 'NONE', ( #13041 ), #1938, .F. ) ;
#8811=LINE ( 'NONE', #6492, #8154 ) ;
#8812=ORIENTED_EDGE ( 'NONE', *, *, #13832, .F. ) ;
#8831=ORIENTED_EDGE ( 'NONE', *, *, #11365, .T. ) ;
#8864=ORIENTED_EDGE ( 'NONE', *, *, #13400, .F. ) ;
#8874=CARTESIAN_POINT ( 'NONE',  ( 470.0000000000000000, -15.00000000000000000, 240.0000000000000284 ) ) ;
#8887=DIRECTION ( 'NONE',  ( -0.000000000000000000, 1.000000000000000000, 0.000000000000000000 ) ) ;
#8888=DIRECTION ( 'NONE',  ( 0.000000000000000000, 1.000000000000000000, 0.000000000000000000 ) ) ;
#8904=FACE_BOUND ( 'NONE', #7837, .T. ) ;
#8938=DIRECTION ( 'NONE',  ( 0.000000000000000000, 0.000000000000000000, 1.000000000000000000 ) ) ;
#8943=CARTESIAN_POINT ( 'NONE',  ( 470.0000000000000000, -15.00000000000000000, 205.0000000000000284 ) ) ;
#8944=CARTESIAN_POINT ( 'NONE',  ( -5.000000000000000888, 8.660254037844390851, 200.0000000000000000 ) ) ;
#8962=AXIS2_PLACEMENT_3D ( 'NONE', #1182, #8888, #10181 ) ;
#8969=AXIS2_PLACEMENT_3D ( 'NONE', #13011, #5256, #8361 ) ;
#8975=AXIS2_PLACEMENT_3D ( 'NONE', #3092, #12007, #2056 ) ;
#8982=FACE_OUTER_BOUND ( 'NONE', #10493, .T. ) ;
#8988=VECTOR ( 'NONE', #8446, 1000.000000000000000 ) ;
#8993=LINE ( 'NONE', #10973, #12711 ) ;
#9000=DIRECTION ( 'NONE',  ( -0.000000000000000000, -0.000000000000000000, 1.000000000000000000 ) ) ;
#9001=ADVANCED_FACE ( 'NONE', ( #6585 ), #11012, .F. ) ;
#9038=CARTESIAN_POINT ( 'NONE',  ( 82.99999999999998579, 8.660254037844390851, 200.0000000000000000 ) ) ;
#9047=ORIENTED_EDGE ( 'NONE', *, *, #3485, .T. ) ;
#9059=CARTESIAN_POINT ( 'NONE',  ( 347.0000000000000000, 8.660254037844390851, 199.9990000000000236 ) ) ;
#9087=ORIENTED_EDGE ( 'NONE', *, *, #6032, .F. ) ;
#9088=EDGE_LOOP ( 'NONE', ( #2308, #718, #14020, #12697 ) ) ;
#9093=MECHANICAL_DESIGN_GEOMETRIC_PRESENTATION_REPRESENTATION('',(#10484),#12107);
#9108=PRESENTATION_STYLE_ASSIGNMENT (( #3669 ) ) ;
#9154=EDGE_LOOP ( 'NONE', ( #13521, #10632, #11511, #5465 ) ) ;
#9162=VERTEX_POINT ( 'NONE', #13025 ) ;
#9163=DIRECTION ( 'NONE',  ( -1.000000000000000000, -0.000000000000000000, -0.000000000000000000 ) ) ;
#9166=DIRECTION ( 'NONE',  ( 0.000000000000000000, -1.000000000000000000, 0.000000000000000000 ) ) ;
#9180=AXIS2_PLACEMENT_3D ( 'NONE', #537, #311, #4778 ) ;
#9192=LINE ( 'NONE', #5074, #1393 ) ;
#9197=FACE_OUTER_BOUND ( 'NONE', #13378, .T. ) ;
#9206=EDGE_CURVE ( 'NONE', #898, #8606, #12951, .T. ) ;
#9223=DIRECTION ( 'NONE',  ( 0.000000000000000000, 1.000000000000000000, 0.000000000000000000 ) ) ;
#9230=EDGE_LOOP ( 'NONE', ( #13505, #8318, #2880, #5182, #2856, #6853 ) ) ;
#9261=DIRECTION ( 'NONE',  ( 0.000000000000000000, -1.000000000000000000, 0.000000000000000000 ) ) ;
#9273=LINE ( 'NONE', #8172, #7318 ) ;
#9290=DIRECTION ( 'NONE',  ( -0.000000000000000000, 0.000000000000000000, 1.000000000000000000 ) ) ;
#9294=VERTEX_POINT ( 'NONE', #5686 ) ;
#9299=DIRECTION ( 'NONE',  ( -1.000000000000000000, 0.000000000000000000, 0.000000000000000000 ) ) ;
#9306=FACE_BOUND ( 'NONE', #2473, .T. ) ;
#9338=CARTESIAN_POINT ( 'NONE',  ( 347.0000000000000000, -8.660254037844389075, 205.0000000000000284 ) ) ;
#9340=DIRECTION ( 'NONE',  ( 0.000000000000000000, -1.000000000000000000, 0.000000000000000000 ) ) ;
#9350=ORIENTED_EDGE ( 'NONE', *, *, #4096, .T. ) ;
#9357=CARTESIAN_POINT ( 'NONE',  ( 53.33333333333330017, -15.00000000000000000, 222.5000000000000853 ) ) ;
#9366=ORIENTED_EDGE ( 'NONE', *, *, #8367, .F. ) ;
#9368=LINE ( 'NONE', #12696, #5053 ) ;
#9371=CARTESIAN_POINT ( 'NONE',  ( 386.6666666666666288, -15.00000000000000000, 222.5000000000000853 ) ) ;
#9377=CARTESIAN_POINT ( 'NONE',  ( -30.00000000000002842, -20.00000000000000000, 240.0000000000000284 ) ) ;
#9383=VERTEX_POINT ( 'NONE', #12086 ) ;
#9385=CARTESIAN_POINT ( 'NONE',  ( -5.000000000000000888, 8.660254037844390851, 205.0000000000000284 ) ) ;
#9400=EDGE_LOOP ( 'NONE', ( #2964, #3396 ) ) ;
#9407=PLANE ( 'NONE',  #13570 ) ;
#9410=AXIS2_PLACEMENT_3D ( 'NONE', #8782, #7612, #10017 ) ;
#9414=DIRECTION ( 'NONE',  ( 0.000000000000000000, -1.000000000000000000, 0.000000000000000000 ) ) ;
#9418=DIRECTION ( 'NONE',  ( 0.000000000000000000, 0.000000000000000000, 1.000000000000000000 ) ) ;
#9433=FACE_OUTER_BOUND ( 'NONE', #3209, .T. ) ;
#9444=FACE_BOUND ( 'NONE', #6164, .T. ) ;
#9451=ORIENTED_EDGE ( 'NONE', *, *, #11365, .F. ) ;
#9477=CARTESIAN_POINT ( 'NONE',  ( 434.9999999999999432, -8.660254037844389075, 200.0000000000000000 ) ) ;
#9488=ADVANCED_FACE ( 'NONE', ( #4899 ), #5981, .F. ) ;
#9497=DIRECTION ( 'NONE',  ( 0.000000000000000000, 1.000000000000000000, 0.000000000000000000 ) ) ;
#9501=ORIENTED_EDGE ( 'NONE', *, *, #8070, .T. ) ;
#9505=LINE ( 'NONE', #10519, #3103 ) ;
#9511=CARTESIAN_POINT ( 'NONE',  ( 136.6666666666666288, -14.99999999999999822, 225.1500000000000625 ) ) ;
#9514=ORIENTED_EDGE ( 'NONE', *, *, #12414, .F. ) ;
#9525=EDGE_CURVE ( 'NONE', #4058, #7268, #8291, .T. ) ;
#9529=DIRECTION ( 'NONE',  ( 1.000000000000000000, 0.000000000000000000, 0.000000000000000000 ) ) ;
#9530=ORIENTED_EDGE ( 'NONE', *, *, #10621, .F. ) ;
#9562=AXIS2_PLACEMENT_3D ( 'NONE', #7289, #5133, #1547 ) ;
#9574=VECTOR ( 'NONE', #10104, 1000.000000000000000 ) ;
#9603=DIRECTION ( 'NONE',  ( -0.000000000000000000, -0.000000000000000000, 1.000000000000000000 ) ) ;
#9617=CARTESIAN_POINT ( 'NONE',  ( 303.3333333333333144, -20.00000000000000000, 222.5000000000000853 ) ) ;
#9620=AXIS2_PLACEMENT_3D ( 'NONE', #14221, #9668, #14081 ) ;
#9621=ORIENTED_EDGE ( 'NONE', *, *, #6640, .F. ) ;
#9635=VECTOR ( 'NONE', #1511, 1000.000000000000000 ) ;
#9640=DIRECTION ( 'NONE',  ( 0.000000000000000000, -1.000000000000000000, 0.000000000000000000 ) ) ;
#9643=FACE_OUTER_BOUND ( 'NONE', #9230, .T. ) ;
#9653=DIRECTION ( 'NONE',  ( 0.000000000000000000, -0.000000000000000000, -1.000000000000000000 ) ) ;
#9658=ADVANCED_FACE ( 'NONE', ( #8707 ), #12119, .F. ) ;
#9664=CIRCLE ( 'NONE', #116, 2.649999999999985700 ) ;
#9668=DIRECTION ( 'NONE',  ( -0.000000000000000000, 0.000000000000000000, -1.000000000000000000 ) ) ;
#9669=AXIS2_PLACEMENT_3D ( 'NONE', #11139, #7923, #5624 ) ;
#9671=CARTESIAN_POINT ( 'NONE',  ( 170.9999999999999716, -8.660254037844389075, 205.0000000000000284 ) ) ;
#9674=ORIENTED_EDGE ( 'NONE', *, *, #5525, .T. ) ;
#9675=LINE ( 'NONE', #725, #2254 ) ;
#9683=EDGE_CURVE ( 'NONE', #3582, #8038, #6194, .T. ) ;
#9686=CARTESIAN_POINT ( 'NONE',  ( 470.0000000000000000, -20.00000000000000000, 240.0000000000000284 ) ) ;
#9688=DIRECTION ( 'NONE',  ( -1.000000000000000000, 0.000000000000000000, 0.000000000000000000 ) ) ;
#9690=VECTOR ( 'NONE', #12448, 1000.000000000000000 ) ;
#9693=LINE ( 'NONE', #6351, #4933 ) ;
#9695=CARTESIAN_POINT ( 'NONE',  ( 93.00000000000000000, 8.660254037844390851, 205.0000000000000284 ) ) ;
#9701=CARTESIAN_POINT ( 'NONE',  ( 53.33333333333330017, -15.00000000000000000, 225.1500000000000625 ) ) ;
#9709=EDGE_CURVE ( 'NONE', #7034, #12519, #11783, .T. ) ;
#9715=DIRECTION ( 'NONE',  ( 0.000000000000000000, -0.000000000000000000, -1.000000000000000000 ) ) ;
#9718=DIRECTION ( 'NONE',  ( -0.000000000000000000, 0.000000000000000000, -1.000000000000000000 ) ) ;
#9722=CARTESIAN_POINT ( 'NONE',  ( -30.00000000000000000, 0.000000000000000000, 205.0000000000000284 ) ) ;
#9725=DIRECTION ( 'NONE',  ( -1.000000000000000000, 0.000000000000000000, -0.000000000000000000 ) ) ;
#9751=FACE_OUTER_BOUND ( 'NONE', #1822, .T. ) ;
#9767=CARTESIAN_POINT ( 'NONE',  ( -30.00000000000002842, -20.00000000000000000, 240.0000000000000284 ) ) ;
#9773=VERTEX_POINT ( 'NONE', #4572 ) ;
#9774=ORIENTED_EDGE ( 'NONE', *, *, #10592, .F. ) ;
#9785=CARTESIAN_POINT ( 'NONE',  ( 93.00000000000000000, -8.660254037844389075, 200.0000000000000000 ) ) ;
#9793=CARTESIAN_POINT ( 'NONE',  ( 4.999999999999999112, 8.660254037844390851, 205.0000000000000284 ) ) ;
#9855=EDGE_LOOP ( 'NONE', ( #11191, #3004, #7423, #13549 ) ) ;
#9863=CIRCLE ( 'NONE', #14252, 2.649999999999985700 ) ;
#9879=DIRECTION ( 'NONE',  ( -0.000000000000000000, 1.000000000000000000, -0.000000000000000000 ) ) ;
#9885=LINE ( 'NONE', #12197, #1543 ) ;
#9888=VECTOR ( 'NONE', #1789, 1000.000000000000000 ) ;
#9894=( NAMED_UNIT ( * ) PLANE_ANGLE_UNIT ( ) SI_UNIT ( $, .RADIAN. ) );
#9902=LINE ( 'NONE', #5680, #9574 ) ;
#9924=CARTESIAN_POINT ( 'NONE',  ( -5.000000000000000888, 8.660254037844390851, 199.9990000000000236 ) ) ;
#9928=VECTOR ( 'NONE', #4406, 1000.000000000000000 ) ;
#9944=CIRCLE ( 'NONE', #8548, 2.649999999999985700 ) ;
#9946=DIRECTION ( 'NONE',  ( -0.000000000000000000, 1.000000000000000000, -0.000000000000000000 ) ) ;
#9955=PLANE ( 'NONE',  #7227 ) ;
#9977=CARTESIAN_POINT ( 'NONE',  ( 181.0000000000000000, -8.660254037844389075, 200.0000000000000000 ) ) ;
#9992=EDGE_CURVE ( 'NONE', #13397, #532, #7163, .T. ) ;
#9998=LINE ( 'NONE', #12312, #11121 ) ;
#10006=CARTESIAN_POINT ( 'NONE',  ( 82.99999999999998579, 8.660254037844390851, 205.0000000000000284 ) ) ;
#10017=DIRECTION ( 'NONE',  ( 0.000000000000000000, 0.000000000000000000, 1.000000000000000000 ) ) ;
#10023=ORIENTED_EDGE ( 'NONE', *, *, #3749, .T. ) ;
#10025=ORIENTED_EDGE ( 'NONE', *, *, #900, .T. ) ;
#10029=FACE_OUTER_BOUND ( 'NONE', #7851, .T. ) ;
#10031=ORIENTED_EDGE ( 'NONE', *, *, #6484, .F. ) ;
#10037=CARTESIAN_POINT ( 'NONE',  ( -30.00000000000002842, -20.00000000000000000, 240.0000000000000284 ) ) ;
#10048=CYLINDRICAL_SURFACE ( 'NONE', #9669, 2.649999999999985700 ) ;
#10066=ORIENTED_EDGE ( 'NONE', *, *, #3329, .F. ) ;
#10085=CARTESIAN_POINT ( 'NONE',  ( 386.6666666666666288, -15.00000000000000000, 219.8500000000001080 ) ) ;
#10091=VERTEX_POINT ( 'NONE', #11292 ) ;
#10096=CARTESIAN_POINT ( 'NONE',  ( 53.33333333333330017, -14.99999999999999822, 222.5000000000000853 ) ) ;
#10104=DIRECTION ( 'NONE',  ( 0.000000000000000000, -1.000000000000000000, 0.000000000000000000 ) ) ;
#10126=FACE_OUTER_BOUND ( 'NONE', #1423, .T. ) ;
#10129=CIRCLE ( 'NONE', #13826, 2.649999999999985700 ) ;
#10157=EDGE_LOOP ( 'NONE', ( #5086, #3350, #3155, #13100 ) ) ;
#10169=CYLINDRICAL_SURFACE ( 'NONE', #12496, 2.649999999999985700 ) ;
#10176=VERTEX_POINT ( 'NONE', #8083 ) ;
#10177=VERTEX_POINT ( 'NONE', #2584 ) ;
#10181=DIRECTION ( 'NONE',  ( 0.000000000000000000, 0.000000000000000000, 1.000000000000000000 ) ) ;
#10182=ADVANCED_FACE ( 'NONE', ( #7004 ), #158, .F. ) ;
#10191=EDGE_CURVE ( 'NONE', #4081, #930, #6795, .T. ) ;
#10192=VERTEX_POINT ( 'NONE', #3887 ) ;
#10206=EDGE_CURVE ( 'NONE', #9383, #7171, #10561, .T. ) ;
#10215=CARTESIAN_POINT ( 'NONE',  ( 82.99999999999998579, -8.660254037844389075, 199.9990000000000236 ) ) ;
#10224=CARTESIAN_POINT ( 'NONE',  ( 434.9999999999999432, 8.660254037844390851, 200.0000000000000000 ) ) ;
#10229=ORIENTED_EDGE ( 'NONE', *, *, #3329, .T. ) ;
#10230=DIRECTION ( 'NONE',  ( -0.000000000000000000, 1.000000000000000000, -0.000000000000000000 ) ) ;
#10235=ORIENTED_EDGE ( 'NONE', *, *, #10293, .F. ) ;
#10240=LINE ( 'NONE', #410, #4847 ) ;
#10246=ORIENTED_EDGE ( 'NONE', *, *, #5525, .F. ) ;
#10257=LINE ( 'NONE', #285, #3417 ) ;
#10275=DIRECTION ( 'NONE',  ( 0.000000000000000000, 0.000000000000000000, 1.000000000000000000 ) ) ;
#10279=ORIENTED_EDGE ( 'NONE', *, *, #3043, .T. ) ;
#10283=FACE_OUTER_BOUND ( 'NONE', #6798, .T. ) ;
#10292=ORIENTED_EDGE ( 'NONE', *, *, #13568, .F. ) ;
#10293=EDGE_CURVE ( 'NONE', #13284, #13567, #4034, .T. ) ;
#10305=DIRECTION ( 'NONE',  ( -0.000000000000000000, 1.000000000000000000, -0.000000000000000000 ) ) ;
#10325=EDGE_CURVE ( 'NONE', #7171, #574, #3757, .T. ) ;
#10327=CARTESIAN_POINT ( 'NONE',  ( 357.0000000000000000, 8.660254037844390851, 200.0000000000000000 ) ) ;
#10344=CARTESIAN_POINT ( 'NONE',  ( 444.9999999999999432, 8.660254037844390851, 205.0000000000000284 ) ) ;
#10347=CIRCLE ( 'NONE', #8962, 2.649999999999985700 ) ;
#10383=DIRECTION ( 'NONE',  ( 1.000000000000000000, 0.000000000000000000, 0.000000000000000000 ) ) ;
#10388=ORIENTED_EDGE ( 'NONE', *, *, #9992, .T. ) ;
#10399=CIRCLE ( 'NONE', #5996, 2.649999999999985700 ) ;
#10402=DIRECTION ( 'NONE',  ( 0.000000000000000000, -0.000000000000000000, -1.000000000000000000 ) ) ;
#10430=EDGE_LOOP ( 'NONE', ( #3307, #6186, #14006, #5915 ) ) ;
#10431=DIRECTION ( 'NONE',  ( -0.000000000000000000, 1.000000000000000000, -0.000000000000000000 ) ) ;
#10433=VECTOR ( 'NONE', #8063, 1000.000000000000000 ) ;
#10448=CARTESIAN_POINT ( 'NONE',  ( -30.00000000000002842, -20.00000000000000000, 240.0000000000000284 ) ) ;
#10455=DIRECTION ( 'NONE',  ( 0.000000000000000000, 0.000000000000000000, -1.000000000000000000 ) ) ;
#10459=CARTESIAN_POINT ( 'NONE',  ( -5.000000000000000888, -8.660254037844389075, 205.0000000000000284 ) ) ;
#10477=CARTESIAN_POINT ( 'NONE',  ( -5.000000000000000888, -8.660254037844389075, 199.9990000000000236 ) ) ;
#10484=STYLED_ITEM ( 'NONE', ( #9108 ), #1760 ) ;
#10493=EDGE_LOOP ( 'NONE', ( #11397, #424, #11025, #8425 ) ) ;
#10500=CARTESIAN_POINT ( 'NONE',  ( 347.0000000000000000, -8.660254037844389075, 199.9990000000000236 ) ) ;
#10501=AXIS2_PLACEMENT_3D ( 'NONE', #13701, #2419, #3840 ) ;
#10508=CARTESIAN_POINT ( 'NONE',  ( 0.000000000000000000, 0.000000000000000000, 0.000000000000000000 ) ) ;
#10519=CARTESIAN_POINT ( 'NONE',  ( 434.9999999999999432, 8.660254037844390851, 205.0000000000000284 ) ) ;
#10527=ORIENTED_EDGE ( 'NONE', *, *, #8747, .F. ) ;
#10529=DIRECTION ( 'NONE',  ( 0.000000000000000000, 0.000000000000000000, -1.000000000000000000 ) ) ;
#10535=VERTEX_POINT ( 'NONE', #4031 ) ;
#10547=APPLICATION_CONTEXT ( 'automotive_design' ) ;
#10556=AXIS2_PLACEMENT_3D ( 'NONE', #2340, #11329, #6759 ) ;
#10561=LINE ( 'NONE', #5205, #11642 ) ;
#10570=LINE ( 'NONE', #13894, #12887 ) ;
#10578=CARTESIAN_POINT ( 'NONE',  ( -5.000000000000000888, -8.660254037844389075, 200.0000000000000000 ) ) ;
#10592=EDGE_CURVE ( 'NONE', #11555, #9162, #1675, .T. ) ;
#10600=EDGE_LOOP ( 'NONE', ( #5248, #12531, #13789, #11457 ) ) ;
#10621=EDGE_CURVE ( 'NONE', #2327, #8720, #9693, .T. ) ;
#10632=ORIENTED_EDGE ( 'NONE', *, *, #7073, .T. ) ;
#10664=CARTESIAN_POINT ( 'NONE',  ( 219.9999999999999716, -20.00000000000000000, 222.5000000000000853 ) ) ;
#10672=VECTOR ( 'NONE', #2219, 1000.000000000000000 ) ;
#10673=VERTEX_POINT ( 'NONE', #9977 ) ;
#10677=DIRECTION ( 'NONE',  ( 0.000000000000000000, -0.000000000000000000, 1.000000000000000000 ) ) ;
#10680=CARTESIAN_POINT ( 'NONE',  ( 470.0000000000000000, 15.00000000000000000, 205.0000000000000284 ) ) ;
#10701=VECTOR ( 'NONE', #5744, 1000.000000000000000 ) ;
#10705=EDGE_CURVE ( 'NONE', #2464, #806, #2060, .T. ) ;
#10729=EDGE_CURVE ( 'NONE', #10177, #13284, #9902, .T. ) ;
#10733=EDGE_CURVE ( 'NONE', #8663, #4316, #8811, .T. ) ;
#10738=EDGE_LOOP ( 'NONE', ( #4011, #10229, #12819, #6807 ) ) ;
#10791=DIRECTION ( 'NONE',  ( 0.000000000000000000, 0.000000000000000000, 1.000000000000000000 ) ) ;
#10793=AXIS2_PLACEMENT_3D ( 'NONE', #1873, #7461, #6303 ) ;
#10800=LINE ( 'NONE', #12824, #9888 ) ;
#10804=DIRECTION ( 'NONE',  ( 1.000000000000000000, 0.000000000000000000, 0.000000000000000000 ) ) ;
#10807=CARTESIAN_POINT ( 'NONE',  ( 181.0000000000000000, 8.660254037844390851, 205.0000000000000284 ) ) ;
#10816=CARTESIAN_POINT ( 'NONE',  ( 219.9999999999999716, -14.99999999999999822, 225.1500000000000625 ) ) ;
#10822=AXIS2_PLACEMENT_3D ( 'NONE', #8613, #831, #13901 ) ;
#10827=ADVANCED_FACE ( 'NONE', ( #3516 ), #8185, .F. ) ;
#10839=DIRECTION ( 'NONE',  ( -1.000000000000000000, 0.000000000000000000, 0.000000000000000000 ) ) ;
#10843=DIRECTION ( 'NONE',  ( 0.000000000000000000, -1.000000000000000000, 0.000000000000000000 ) ) ;
#10871=VECTOR ( 'NONE', #9640, 1000.000000000000000 ) ;
#10875=DIRECTION ( 'NONE',  ( 0.000000000000000000, -1.000000000000000000, 0.000000000000000000 ) ) ;
#10892=CARTESIAN_POINT ( 'NONE',  ( -30.00000000000002842, -15.00000000000000000, 240.0000000000000284 ) ) ;
#10904=EDGE_LOOP ( 'NONE', ( #7694, #7142, #8812, #3579 ) ) ;
#10908=EDGE_CURVE ( 'NONE', #4652, #4058, #9505, .T. ) ;
#10917=AXIS2_PLACEMENT_3D ( 'NONE', #7928, #1939, #5554 ) ;
#10923=ADVANCED_FACE ( 'NONE', ( #9433 ), #13772, .F. ) ;
#10935=EDGE_CURVE ( 'NONE', #8786, #14065, #6236, .T. ) ;
#10964=DIRECTION ( 'NONE',  ( -0.000000000000000000, 1.000000000000000000, 0.000000000000000000 ) ) ;
#10973=CARTESIAN_POINT ( 'NONE',  ( 82.99999999999998579, 8.660254037844390851, 200.0000000000000000 ) ) ;
#11007=AXIS2_PLACEMENT_3D ( 'NONE', #9377, #6332, #3000 ) ;
#11009=ORIENTED_EDGE ( 'NONE', *, *, #10325, .F. ) ;
#11012=PLANE ( 'NONE',  #3185 ) ;
#11015=AXIS2_PLACEMENT_3D ( 'NONE', #7832, #12476, #6819 ) ;
#11025=ORIENTED_EDGE ( 'NONE', *, *, #2163, .F. ) ;
#11070=CARTESIAN_POINT ( 'NONE',  ( 470.0000000000000000, 15.00000000000000000, 200.0000000000000000 ) ) ;
#11077=CARTESIAN_POINT ( 'NONE',  ( 357.0000000000000000, 8.660254037844390851, 205.0000000000000284 ) ) ;
#11082=EDGE_LOOP ( 'NONE', ( #1692, #6608, #1949, #964 ) ) ;
#11112=DIRECTION ( 'NONE',  ( -0.000000000000000000, 1.000000000000000000, -0.000000000000000000 ) ) ;
#11119=EDGE_CURVE ( 'NONE', #3734, #2838, #3609, .T. ) ;
#11121=VECTOR ( 'NONE', #13184, 1000.000000000000000 ) ;
#11139=CARTESIAN_POINT ( 'NONE',  ( 136.6666666666666288, -15.00000000000000000, 222.5000000000000853 ) ) ;
#11142=EDGE_CURVE ( 'NONE', #2517, #2327, #12462, .T. ) ;
#11147=VECTOR ( 'NONE', #970, 1000.000000000000000 ) ;
#11160=ORIENTED_EDGE ( 'NONE', *, *, #1897, .T. ) ;
#11175=VECTOR ( 'NONE', #621, 1000.000000000000000 ) ;
#11189=VERTEX_POINT ( 'NONE', #12385 ) ;
#11191=ORIENTED_EDGE ( 'NONE', *, *, #6565, .T. ) ;
#11194=DIRECTION ( 'NONE',  ( -0.000000000000000000, -0.000000000000000000, 1.000000000000000000 ) ) ;
#11202=AXIS2_PLACEMENT_3D ( 'NONE', #2756, #549, #9290 ) ;
#11215=DIRECTION ( 'NONE',  ( -0.000000000000000000, 1.000000000000000000, -0.000000000000000000 ) ) ;
#11232=ADVANCED_FACE ( 'NONE', ( #8982 ), #5711, .F. ) ;
#11234=ORIENTED_EDGE ( 'NONE', *, *, #9525, .T. ) ;
#11249=ORIENTED_EDGE ( 'NONE', *, *, #2089, .T. ) ;
#11259=DIRECTION ( 'NONE',  ( 0.000000000000000000, 0.000000000000000000, 1.000000000000000000 ) ) ;
#11262=EDGE_CURVE ( 'NONE', #5823, #4652, #9192, .T. ) ;
#11271=ORIENTED_EDGE ( 'NONE', *, *, #10935, .T. ) ;
#11292=CARTESIAN_POINT ( 'NONE',  ( 386.6666666666666288, -20.00000000000000000, 219.8500000000001080 ) ) ;
#11306=DIRECTION ( 'NONE',  ( 0.000000000000000000, 0.000000000000000000, 1.000000000000000000 ) ) ;
#11314=VECTOR ( 'NONE', #730, 1000.000000000000000 ) ;
#11315=FACE_OUTER_BOUND ( 'NONE', #12745, .T. ) ;
#11322=FACE_OUTER_BOUND ( 'NONE', #10600, .T. ) ;
#11329=DIRECTION ( 'NONE',  ( -1.000000000000000000, -0.000000000000000000, 0.000000000000000000 ) ) ;
#11334=DIRECTION ( 'NONE',  ( 1.000000000000000000, 0.000000000000000000, 0.000000000000000000 ) ) ;
#11365=EDGE_CURVE ( 'NONE', #9162, #10535, #2664, .T. ) ;
#11372=DIRECTION ( 'NONE',  ( 0.000000000000000000, 1.000000000000000000, 0.000000000000000000 ) ) ;
#11375=VECTOR ( 'NONE', #12964, 1000.000000000000000 ) ;
#11397=ORIENTED_EDGE ( 'NONE', *, *, #10293, .T. ) ;
#11410=ORIENTED_EDGE ( 'NONE', *, *, #4998, .F. ) ;
#11420=DIRECTION ( 'NONE',  ( -0.000000000000000000, -0.000000000000000000, 1.000000000000000000 ) ) ;
#11432=CARTESIAN_POINT ( 'NONE',  ( 53.33333333333330017, -15.00000000000000000, 222.5000000000000853 ) ) ;
#11438=EDGE_CURVE ( 'NONE', #3406, #6981, #4265, .T. ) ;
#11447=CARTESIAN_POINT ( 'NONE',  ( 386.6666666666666288, -20.00000000000000000, 225.1500000000000625 ) ) ;
#11454=CYLINDRICAL_SURFACE ( 'NONE', #6703, 2.649999999999985700 ) ;
#11457=ORIENTED_EDGE ( 'NONE', *, *, #10206, .F. ) ;
#11472=CARTESIAN_POINT ( 'NONE',  ( 470.0000000000000000, -15.00000000000000000, 240.0000000000000284 ) ) ;
#11473=EDGE_CURVE ( 'NONE', #806, #5643, #8540, .T. ) ;
#11477=CIRCLE ( 'NONE', #11015, 2.649999999999985700 ) ;
#11489=AXIS2_PLACEMENT_3D ( 'NONE', #9722, #13110, #14125 ) ;
#11511=ORIENTED_EDGE ( 'NONE', *, *, #13158, .T. ) ;
#11541=VECTOR ( 'NONE', #427, 1000.000000000000000 ) ;
#11544=FACE_OUTER_BOUND ( 'NONE', #8350, .T. ) ;
#11555=VERTEX_POINT ( 'NONE', #2368 ) ;
#11558=DIRECTION ( 'NONE',  ( -1.000000000000000000, -0.000000000000000000, -0.000000000000000000 ) ) ;
#11559=CARTESIAN_POINT ( 'NONE',  ( 0.000000000000000000, 15.00000000000000000, 200.0000000000000000 ) ) ;
#11573=CARTESIAN_POINT ( 'NONE',  ( 170.9999999999999716, -8.660254037844389075, 199.9990000000000236 ) ) ;
#11581=CARTESIAN_POINT ( 'NONE',  ( 136.6666666666666288, -15.00000000000000000, 219.8500000000001080 ) ) ;
#11594=CARTESIAN_POINT ( 'NONE',  ( 181.0000000000000000, 8.660254037844390851, 199.9990000000000236 ) ) ;
#11596=VECTOR ( 'NONE', #11215, 1000.000000000000000 ) ;
#11605=DIRECTION ( 'NONE',  ( 1.000000000000000000, 0.000000000000000000, 0.000000000000000000 ) ) ;
#11642=VECTOR ( 'NONE', #13885, 1000.000000000000000 ) ;
#11651=AXIS2_PLACEMENT_3D ( 'NONE', #9617, #3020, #11865 ) ;
#11670=FACE_BOUND ( 'NONE', #5580, .T. ) ;
#11695=FACE_OUTER_BOUND ( 'NONE', #3722, .T. ) ;
#11723=DIRECTION ( 'NONE',  ( -0.000000000000000000, 1.000000000000000000, -0.000000000000000000 ) ) ;
#11728=EDGE_CURVE ( 'NONE', #1332, #574, #441, .T. ) ;
#11740=CARTESIAN_POINT ( 'NONE',  ( 0.000000000000000000, 15.00000000000000000, 205.0000000000000284 ) ) ;
#11765=AXIS2_PLACEMENT_3D ( 'NONE', #12375, #4696, #2371 ) ;
#11783=LINE ( 'NONE', #5197, #471 ) ;
#11821=PLANE ( 'NONE',  #10793 ) ;
#11827=DIRECTION ( 'NONE',  ( -1.000000000000000000, 0.000000000000000000, 0.000000000000000000 ) ) ;
#11828=ORIENTED_EDGE ( 'NONE', *, *, #11262, .T. ) ;
#11839=EDGE_CURVE ( 'NONE', #5456, #532, #13085, .T. ) ;
#11844=ORIENTED_EDGE ( 'NONE', *, *, #340, .F. ) ;
#11845=FACE_BOUND ( 'NONE', #2059, .T. ) ;
#11865=DIRECTION ( 'NONE',  ( 0.000000000000000000, 0.000000000000000000, 1.000000000000000000 ) ) ;
#11890=EDGE_CURVE ( 'NONE', #14065, #2517, #2876, .T. ) ;
#11893=LINE ( 'NONE', #12974, #13392 ) ;
#11897=CARTESIAN_POINT ( 'NONE',  ( 219.9999999999999716, -14.99999999999999822, 219.8500000000001080 ) ) ;
#11902=CARTESIAN_POINT ( 'NONE',  ( 303.3333333333333144, -14.99999999999999822, 222.5000000000000853 ) ) ;
#11906=EDGE_CURVE ( 'NONE', #9162, #11555, #9664, .T. ) ;
#11919=CARTESIAN_POINT ( 'NONE',  ( 136.6666666666666288, -15.00000000000000000, 225.1500000000000625 ) ) ;
#11922=EDGE_CURVE ( 'NONE', #4821, #4081, #590, .T. ) ;
#11939=DIRECTION ( 'NONE',  ( -0.000000000000000000, 1.000000000000000000, -0.000000000000000000 ) ) ;
#11941=VECTOR ( 'NONE', #10230, 1000.000000000000000 ) ;
#11944=ORIENTED_EDGE ( 'NONE', *, *, #11839, .F. ) ;
#11965=VERTEX_POINT ( 'NONE', #1921 ) ;
#12007=DIRECTION ( 'NONE',  ( 0.000000000000000000, 1.000000000000000000, 0.000000000000000000 ) ) ;
#12010=EDGE_LOOP ( 'NONE', ( #12192, #13157, #10527, #4578 ) ) ;
#12031=CARTESIAN_POINT ( 'NONE',  ( 470.0000000000000000, -20.00000000000000000, 200.0000000000000000 ) ) ;
#12053=CARTESIAN_POINT ( 'NONE',  ( 470.0000000000000000, -20.00000000000000000, 240.0000000000000284 ) ) ;
#12056=CARTESIAN_POINT ( 'NONE',  ( 434.9999999999999432, 8.660254037844390851, 205.0000000000000284 ) ) ;
#12066=ORIENTED_EDGE ( 'NONE', *, *, #9992, .F. ) ;
#12086=CARTESIAN_POINT ( 'NONE',  ( 219.9999999999999716, -20.00000000000000000, 225.1500000000000625 ) ) ;
#12096=ORIENTED_EDGE ( 'NONE', *, *, #14198, .T. ) ;
#12107=( GEOMETRIC_REPRESENTATION_CONTEXT ( 3 ) GLOBAL_UNCERTAINTY_ASSIGNED_CONTEXT ( ( #2041 ) ) GLOBAL_UNIT_ASSIGNED_CONTEXT ( ( #8000, #7002, #5910 ) ) REPRESENTATION_CONTEXT ( 'NONE', 'WORKASPACE' ) );
#12119=CYLINDRICAL_SURFACE ( 'NONE', #6537, 2.649999999999985700 ) ;
#12129=EDGE_LOOP ( 'NONE', ( #4422, #12569, #9621, #1472 ) ) ;
#12140=VERTEX_POINT ( 'NONE', #11070 ) ;
#12154=EDGE_CURVE ( 'NONE', #4579, #12140, #4466, .T. ) ;
#12161=CARTESIAN_POINT ( 'NONE',  ( 386.6666666666666288, -14.99999999999999822, 222.5000000000000853 ) ) ;
#12165=DIRECTION ( 'NONE',  ( 0.000000000000000000, -1.000000000000000000, 0.000000000000000000 ) ) ;
#12167=AXIS2_PLACEMENT_3D ( 'NONE', #6091, #6234, #8254 ) ;
#12192=ORIENTED_EDGE ( 'NONE', *, *, #13832, .T. ) ;
#12194=VECTOR ( 'NONE', #3897, 1000.000000000000000 ) ;
#12197=CARTESIAN_POINT ( 'NONE',  ( 269.0000000000000000, 8.660254037844390851, 199.9990000000000236 ) ) ;
#12200=FACE_OUTER_BOUND ( 'NONE', #1462, .T. ) ;
#12207=AXIS2_PLACEMENT_3D ( 'NONE', #6842, #7987, #2356 ) ;
#12232=VECTOR ( 'NONE', #12948, 1000.000000000000000 ) ;
#12264=CARTESIAN_POINT ( 'NONE',  ( 82.99999999999998579, 8.660254037844390851, 199.9990000000000236 ) ) ;
#12276=PLANE ( 'NONE',  #10556 ) ;
#12286=VECTOR ( 'NONE', #11605, 1000.000000000000000 ) ;
#12292=PLANE ( 'NONE',  #12207 ) ;
#12295=VECTOR ( 'NONE', #4745, 1000.000000000000000 ) ;
#12301=EDGE_CURVE ( 'NONE', #514, #8786, #13728, .T. ) ;
#12312=CARTESIAN_POINT ( 'NONE',  ( 470.0000000000000000, -20.00000000000000000, 240.0000000000000284 ) ) ;
#12332=ORIENTED_EDGE ( 'NONE', *, *, #2655, .T. ) ;
#12333=COLOUR_RGB ( '',0.8941176470588234615, 0.8941176470588234615, 0.8941176470588234615 ) ;
#12337=DIRECTION ( 'NONE',  ( 0.000000000000000000, 1.000000000000000000, 0.000000000000000000 ) ) ;
#12350=LINE ( 'NONE', #1308, #10701 ) ;
#12363=CARTESIAN_POINT ( 'NONE',  ( 470.0000000000000000, 0.000000000000000000, 200.0000000000000000 ) ) ;
#12370=LINE ( 'NONE', #12511, #7979 ) ;
#12372=( NAMED_UNIT ( * ) SI_UNIT ( $, .STERADIAN. ) SOLID_ANGLE_UNIT ( ) );
#12375=CARTESIAN_POINT ( 'NONE',  ( 0.000000000000000000, -15.00000000000000000, 0.000000000000000000 ) ) ;
#12377=ORIENTED_EDGE ( 'NONE', *, *, #6565, .F. ) ;
#12385=CARTESIAN_POINT ( 'NONE',  ( 259.0000000000000000, 8.660254037844390851, 200.0000000000000000 ) ) ;
#12391=DIRECTION ( 'NONE',  ( 1.000000000000000000, 0.000000000000000000, 0.000000000000000000 ) ) ;
#12414=EDGE_CURVE ( 'NONE', #11189, #6109, #9675, .T. ) ;
#12418=ORIENTED_EDGE ( 'NONE', *, *, #13053, .T. ) ;
#12423=AXIS2_PLACEMENT_3D ( 'NONE', #12161, #13654, #8141 ) ;
#12425=CARTESIAN_POINT ( 'NONE',  ( 82.99999999999998579, -8.660254037844389075, 200.0000000000000000 ) ) ;
#12448=DIRECTION ( 'NONE',  ( -0.000000000000000000, -0.000000000000000000, 1.000000000000000000 ) ) ;
#12462=LINE ( 'NONE', #10006, #2331 ) ;
#12471=LINE ( 'NONE', #3767, #8013 ) ;
#12476=DIRECTION ( 'NONE',  ( -0.000000000000000000, 1.000000000000000000, -0.000000000000000000 ) ) ;
#12492=VECTOR ( 'NONE', #12165, 1000.000000000000000 ) ;
#12496=AXIS2_PLACEMENT_3D ( 'NONE', #9371, #6903, #7908 ) ;
#12502=EDGE_CURVE ( 'NONE', #8482, #4614, #2860, .T. ) ;
#12511=CARTESIAN_POINT ( 'NONE',  ( 347.0000000000000000, 8.660254037844390851, 205.0000000000000284 ) ) ;
#12518=LINE ( 'NONE', #1476, #2742 ) ;
#12519=VERTEX_POINT ( 'NONE', #5665 ) ;
#12520=AXIS2_PLACEMENT_3D ( 'NONE', #4999, #5080, #7308 ) ;
#12531=ORIENTED_EDGE ( 'NONE', *, *, #11728, .T. ) ;
#12541=STYLED_ITEM('',(#14396),#3714);
#12560=FACE_OUTER_BOUND ( 'NONE', #9088, .T. ) ;
#12569=ORIENTED_EDGE ( 'NONE', *, *, #13490, .F. ) ;
#12594=LINE ( 'NONE', #4919, #5476 ) ;
#12601=EDGE_CURVE ( 'NONE', #12519, #6497, #9885, .T. ) ;
#12602=DIRECTION ( 'NONE',  ( -1.000000000000000000, -0.000000000000000000, -0.000000000000000000 ) ) ;
#12605=CYLINDRICAL_SURFACE ( 'NONE', #5571, 2.649999999999985700 ) ;
#12607=DIRECTION ( 'NONE',  ( 0.000000000000000000, -1.000000000000000000, 0.000000000000000000 ) ) ;
#12621=ORIENTED_EDGE ( 'NONE', *, *, #13400, .T. ) ;
#12626=CARTESIAN_POINT ( 'NONE',  ( 434.9999999999999432, 8.660254037844390851, 199.9990000000000236 ) ) ;
#12670=VECTOR ( 'NONE', #11194, 1000.000000000000000 ) ;
#12672=LINE ( 'NONE', #3903, #4560 ) ;
#12687=VERTEX_POINT ( 'NONE', #10448 ) ;
#12696=CARTESIAN_POINT ( 'NONE',  ( 259.0000000000000000, 8.660254037844390851, 200.0000000000000000 ) ) ;
#12697=ORIENTED_EDGE ( 'NONE', *, *, #1250, .F. ) ;
#12711=VECTOR ( 'NONE', #13409, 1000.000000000000000 ) ;
#12740=DIRECTION ( 'NONE',  ( -0.000000000000000000, -0.000000000000000000, 1.000000000000000000 ) ) ;
#12741=AXIS2_PLACEMENT_3D ( 'NONE', #6217, #6074, #7018 ) ;
#12745=EDGE_LOOP ( 'NONE', ( #5414, #2921, #5050, #10025 ) ) ;
#12752=FACE_BOUND ( 'NONE', #1156, .T. ) ;
#12766=DIRECTION ( 'NONE',  ( -0.000000000000000000, 1.000000000000000000, -0.000000000000000000 ) ) ;
#12767=ORIENTED_EDGE ( 'NONE', *, *, #4268, .T. ) ;
#12773=FACE_BOUND ( 'NONE', #1525, .T. ) ;
#12806=DIRECTION ( 'NONE',  ( -0.000000000000000000, 1.000000000000000000, -0.000000000000000000 ) ) ;
#12809=DIRECTION ( 'NONE',  ( 0.000000000000000000, 1.000000000000000000, 0.000000000000000000 ) ) ;
#12814=EDGE_CURVE ( 'NONE', #4081, #5823, #5790, .T. ) ;
#12819=ORIENTED_EDGE ( 'NONE', *, *, #6119, .F. ) ;
#12824=CARTESIAN_POINT ( 'NONE',  ( 82.99999999999998579, 8.660254037844390851, 199.9990000000000236 ) ) ;
#12827=DIRECTION ( 'NONE',  ( -1.000000000000000000, 0.000000000000000000, 0.000000000000000000 ) ) ;
#12855=VERTEX_POINT ( 'NONE', #8336 ) ;
#12861=DIRECTION ( 'NONE',  ( 0.000000000000000000, 0.000000000000000000, 1.000000000000000000 ) ) ;
#12864=VERTEX_POINT ( 'NONE', #633 ) ;
#12885=EDGE_CURVE ( 'NONE', #10535, #2842, #373, .T. ) ;
#12887=VECTOR ( 'NONE', #12740, 1000.000000000000000 ) ;
#12897=CARTESIAN_POINT ( 'NONE',  ( 444.9999999999999432, 8.660254037844390851, 199.9990000000000236 ) ) ;
#12919=PLANE ( 'NONE',  #7926 ) ;
#12926=PLANE ( 'NONE',  #11007 ) ;
#12940=CARTESIAN_POINT ( 'NONE',  ( 4.999999999999999112, -8.660254037844389075, 205.0000000000000284 ) ) ;
#12946=EDGE_CURVE ( 'NONE', #13937, #6309, #7397, .T. ) ;
#12948=DIRECTION ( 'NONE',  ( 1.000000000000000000, 0.000000000000000000, 0.000000000000000000 ) ) ;
#12951=LINE ( 'NONE', #9701, #7670 ) ;
#12964=DIRECTION ( 'NONE',  ( -1.000000000000000000, 0.000000000000000000, 0.000000000000000000 ) ) ;
#12972=ADVANCED_FACE ( 'NONE', ( #2221, #3533, #6651, #8904, #13316, #10126 ), #89, .T. ) ;
#12974=CARTESIAN_POINT ( 'NONE',  ( 259.0000000000000000, -8.660254037844389075, 205.0000000000000284 ) ) ;
#12990=CARTESIAN_POINT ( 'NONE',  ( 434.9999999999999432, -8.660254037844389075, 205.0000000000000284 ) ) ;
#12994=VECTOR ( 'NONE', #7886, 1000.000000000000000 ) ;
#12996=LINE ( 'NONE', #2995, #2116 ) ;
#13011=CARTESIAN_POINT ( 'NONE',  ( 82.99999999999998579, 8.660254037844390851, 199.9990000000000236 ) ) ;
#13014=CARTESIAN_POINT ( 'NONE',  ( 181.0000000000000000, -8.660254037844389075, 205.0000000000000284 ) ) ;
#13020=ORIENTED_EDGE ( 'NONE', *, *, #7570, .T. ) ;
#13025=CARTESIAN_POINT ( 'NONE',  ( 303.3333333333333144, -20.00000000000000000, 219.8500000000001080 ) ) ;
#13032=ORIENTED_EDGE ( 'NONE', *, *, #9709, .F. ) ;
#13036=CARTESIAN_POINT ( 'NONE',  ( -30.00000000000000000, 0.000000000000000000, 205.0000000000000284 ) ) ;
#13041=FACE_OUTER_BOUND ( 'NONE', #784, .T. ) ;
#13053=EDGE_CURVE ( 'NONE', #2464, #5376, #231, .T. ) ;
#13058=FACE_OUTER_BOUND ( 'NONE', #12010, .T. ) ;
#13067=LINE ( 'NONE', #11919, #13304 ) ;
#13068=ORIENTED_EDGE ( 'NONE', *, *, #8265, .F. ) ;
#13085=LINE ( 'NONE', #2945, #6412 ) ;
#13100=ORIENTED_EDGE ( 'NONE', *, *, #1854, .F. ) ;
#13110=DIRECTION ( 'NONE',  ( 1.000000000000000000, 0.000000000000000000, -0.000000000000000000 ) ) ;
#13112=ORIENTED_EDGE ( 'NONE', *, *, #1155, .F. ) ;
#13133=ORIENTED_EDGE ( 'NONE', *, *, #6343, .T. ) ;
#13135=ORIENTED_EDGE ( 'NONE', *, *, #2637, .F. ) ;
#13153=PLANE ( 'NONE',  #5114 ) ;
#13157=ORIENTED_EDGE ( 'NONE', *, *, #4426, .T. ) ;
#13158=EDGE_CURVE ( 'NONE', #10673, #13397, #12518, .T. ) ;
#13164=ORIENTED_EDGE ( 'NONE', *, *, #6172, .F. ) ;
#13184=DIRECTION ( 'NONE',  ( 0.000000000000000000, 0.000000000000000000, -1.000000000000000000 ) ) ;
#13188=FACE_OUTER_BOUND ( 'NONE', #13366, .T. ) ;
#13201=DIRECTION ( 'NONE',  ( -0.000000000000000000, -0.000000000000000000, 1.000000000000000000 ) ) ;
#13212=DIRECTION ( 'NONE',  ( 0.000000000000000000, 0.000000000000000000, 1.000000000000000000 ) ) ;
#13228=EDGE_CURVE ( 'NONE', #12687, #3582, #14029, .T. ) ;
#13229=EDGE_CURVE ( 'NONE', #10176, #5679, #4103, .T. ) ;
#13236=ORIENTED_EDGE ( 'NONE', *, *, #10206, .T. ) ;
#13242=ORIENTED_EDGE ( 'NONE', *, *, #1350, .F. ) ;
#13269=CARTESIAN_POINT ( 'NONE',  ( 136.6666666666666288, -20.00000000000000000, 219.8500000000001080 ) ) ;
#13284=VERTEX_POINT ( 'NONE', #5549 ) ;
#13285=DIRECTION ( 'NONE',  ( -0.000000000000000000, -0.000000000000000000, 1.000000000000000000 ) ) ;
#13288=DIRECTION ( 'NONE',  ( -0.000000000000000000, 1.000000000000000000, -0.000000000000000000 ) ) ;
#13294=ORIENTED_EDGE ( 'NONE', *, *, #14212, .T. ) ;
#13304=VECTOR ( 'NONE', #6610, 1000.000000000000000 ) ;
#13316=FACE_BOUND ( 'NONE', #352, .T. ) ;
#13317=ORIENTED_EDGE ( 'NONE', *, *, #12885, .T. ) ;
#13329=ORIENTED_EDGE ( 'NONE', *, *, #11922, .T. ) ;
#13332=LINE ( 'NONE', #7679, #13565 ) ;
#13345=CARTESIAN_POINT ( 'NONE',  ( -30.00000000000002842, -15.00000000000000000, 240.0000000000000284 ) ) ;
#13352=CARTESIAN_POINT ( 'NONE',  ( 259.0000000000000000, -8.660254037844389075, 199.9990000000000236 ) ) ;
#13366=EDGE_LOOP ( 'NONE', ( #11271, #3812, #9087, #5367 ) ) ;
#13375=CARTESIAN_POINT ( 'NONE',  ( 53.33333333333330017, -15.00000000000000000, 219.8500000000001080 ) ) ;
#13378=EDGE_LOOP ( 'NONE', ( #6041, #521, #13236, #629 ) ) ;
#13392=VECTOR ( 'NONE', #10804, 1000.000000000000000 ) ;
#13397=VERTEX_POINT ( 'NONE', #3726 ) ;
#13400=EDGE_CURVE ( 'NONE', #12140, #1151, #2571, .T. ) ;
#13409=DIRECTION ( 'NONE',  ( -1.000000000000000000, 0.000000000000000000, 0.000000000000000000 ) ) ;
#13425=DIRECTION ( 'NONE',  ( -0.000000000000000000, 1.000000000000000000, -0.000000000000000000 ) ) ;
#13441=VECTOR ( 'NONE', #176, 1000.000000000000000 ) ;
#13447=DIRECTION ( 'NONE',  ( -1.000000000000000000, -0.000000000000000000, -0.000000000000000000 ) ) ;
#13467=EDGE_LOOP ( 'NONE', ( #3704, #6017, #3136, #5788 ) ) ;
#13473=PLANE ( 'NONE',  #4360 ) ;
#13485=ORIENTED_EDGE ( 'NONE', *, *, #7618, .F. ) ;
#13490=EDGE_CURVE ( 'NONE', #6568, #3844, #507, .T. ) ;
#13493=ORIENTED_EDGE ( 'NONE', *, *, #6032, .T. ) ;
#13502=ORIENTED_EDGE ( 'NONE', *, *, #8167, .T. ) ;
#13503=VERTEX_POINT ( 'NONE', #13511 ) ;
#13505=ORIENTED_EDGE ( 'NONE', *, *, #7562, .T. ) ;
#13510=CARTESIAN_POINT ( 'NONE',  ( 269.0000000000000000, 8.660254037844390851, 205.0000000000000284 ) ) ;
#13511=CARTESIAN_POINT ( 'NONE',  ( 82.99999999999998579, 8.660254037844390851, 200.0000000000000000 ) ) ;
#13521=ORIENTED_EDGE ( 'NONE', *, *, #10729, .T. ) ;
#13534=VECTOR ( 'NONE', #3429, 1000.000000000000000 ) ;
#13549=ORIENTED_EDGE ( 'NONE', *, *, #3576, .F. ) ;
#13565=VECTOR ( 'NONE', #5441, 1000.000000000000000 ) ;
#13567=VERTEX_POINT ( 'NONE', #797 ) ;
#13568=EDGE_CURVE ( 'NONE', #4587, #4579, #4086, .T. ) ;
#13570=AXIS2_PLACEMENT_3D ( 'NONE', #13819, #13680, #6682 ) ;
#13572=LINE ( 'NONE', #3651, #10433 ) ;
#13573=VECTOR ( 'NONE', #5862, 1000.000000000000000 ) ;
#13577=LINE ( 'NONE', #3657, #5717 ) ;
#13581=ADVANCED_FACE ( 'NONE', ( #9751 ), #4162, .F. ) ;
#13594=SURFACE_STYLE_FILL_AREA ( #227 ) ;
#13612=ORIENTED_EDGE ( 'NONE', *, *, #2334, .F. ) ;
#13614=CARTESIAN_POINT ( 'NONE',  ( 444.9999999999999432, -8.660254037844389075, 199.9990000000000236 ) ) ;
#13618=CARTESIAN_POINT ( 'NONE',  ( 0.000000000000000000, 15.00000000000000000, 205.0000000000000284 ) ) ;
#13624=DIRECTION ( 'NONE',  ( -0.000000000000000000, 1.000000000000000000, -0.000000000000000000 ) ) ;
#13634=DIRECTION ( 'NONE',  ( -1.000000000000000000, 0.000000000000000000, 0.000000000000000000 ) ) ;
#13648=VECTOR ( 'NONE', #11334, 1000.000000000000000 ) ;
#13654=DIRECTION ( 'NONE',  ( -0.000000000000000000, 1.000000000000000000, -0.000000000000000000 ) ) ;
#13657=PRODUCT_DEFINITION ( 'UNKNOWN', '', #6320, #829 ) ;
#13668=SHAPE_REPRESENTATION_RELATIONSHIP ( 'NONE' , 'NONE' ,  #3832, #1760 ) ;
#13670=EDGE_CURVE ( 'NONE', #7167, #7113, #10129, .T. ) ;
#13680=DIRECTION ( 'NONE',  ( -1.000000000000000000, 0.000000000000000000, -0.000000000000000000 ) ) ;
#13701=CARTESIAN_POINT ( 'NONE',  ( 434.9999999999999432, 8.660254037844390851, 199.9990000000000236 ) ) ;
#13710=PLANE ( 'NONE',  #4571 ) ;
#13715=DIRECTION ( 'NONE',  ( 0.000000000000000000, -0.000000000000000000, 1.000000000000000000 ) ) ;
#13728=LINE ( 'NONE', #12425, #6420 ) ;
#13751=PLANE ( 'NONE',  #8005 ) ;
#13757=PLANE ( 'NONE',  #9180 ) ;
#13772=PLANE ( 'NONE',  #10501 ) ;
#13788=ORIENTED_EDGE ( 'NONE', *, *, #1897, .F. ) ;
#13789=ORIENTED_EDGE ( 'NONE', *, *, #308, .T. ) ;
#13805=ORIENTED_EDGE ( 'NONE', *, *, #8070, .F. ) ;
#13818=CARTESIAN_POINT ( 'NONE',  ( 181.0000000000000000, -8.660254037844389075, 199.9990000000000236 ) ) ;
#13819=CARTESIAN_POINT ( 'NONE',  ( 347.0000000000000000, 8.660254037844390851, 199.9990000000000236 ) ) ;
#13826=AXIS2_PLACEMENT_3D ( 'NONE', #4383, #7631, #1233 ) ;
#13832=EDGE_CURVE ( 'NONE', #9294, #9773, #4520, .T. ) ;
#13841=ORIENTED_EDGE ( 'NONE', *, *, #12601, .F. ) ;
#13852=ADVANCED_FACE ( 'NONE', ( #2551 ), #7180, .F. ) ;
#13857=DIRECTION ( 'NONE',  ( 1.000000000000000000, 0.000000000000000000, 0.000000000000000000 ) ) ;
#13868=ORIENTED_EDGE ( 'NONE', *, *, #4975, .F. ) ;
#13885=DIRECTION ( 'NONE',  ( -0.000000000000000000, 1.000000000000000000, -0.000000000000000000 ) ) ;
#13894=CARTESIAN_POINT ( 'NONE',  ( 357.0000000000000000, 8.660254037844390851, 199.9990000000000236 ) ) ;
#13901=DIRECTION ( 'NONE',  ( 0.000000000000000000, 0.000000000000000000, 1.000000000000000000 ) ) ;
#13912=FACE_OUTER_BOUND ( 'NONE', #8066, .T. ) ;
#13921=MECHANICAL_DESIGN_GEOMETRIC_PRESENTATION_REPRESENTATION('',(#12541),#4413);
#13935=EDGE_CURVE ( 'NONE', #12519, #11189, #9368, .T. ) ;
#13937=VERTEX_POINT ( 'NONE', #4877 ) ;
#13939=LINE ( 'NONE', #9671, #7649 ) ;
#14006=ORIENTED_EDGE ( 'NONE', *, *, #8167, .F. ) ;
#14020=ORIENTED_EDGE ( 'NONE', *, *, #13228, .F. ) ;
#14029=LINE ( 'NONE', #9767, #12232 ) ;
#14039=AXIS2_PLACEMENT_3D ( 'NONE', #10508, #9418, #5077 ) ;
#14043=AXIS2_PLACEMENT_3D ( 'NONE', #6748, #2659, #10275 ) ;
#14063=PLANE ( 'NONE',  #7863 ) ;
#14065=VERTEX_POINT ( 'NONE', #6315 ) ;
#14068=DIRECTION ( 'NONE',  ( 0.000000000000000000, -1.000000000000000000, 0.000000000000000000 ) ) ;
#14071=ORIENTED_EDGE ( 'NONE', *, *, #12154, .F. ) ;
#14081=DIRECTION ( 'NONE',  ( -1.000000000000000000, 0.000000000000000000, 0.000000000000000000 ) ) ;
#14120=CARTESIAN_POINT ( 'NONE',  ( 386.6666666666666288, -14.99999999999999822, 225.1500000000000625 ) ) ;
#14125=DIRECTION ( 'NONE',  ( -0.000000000000000000, 0.000000000000000000, -1.000000000000000000 ) ) ;
#14133=ORIENTED_EDGE ( 'NONE', *, *, #6119, .T. ) ;
#14136=EDGE_LOOP ( 'NONE', ( #10388, #11160, #6396, #3796 ) ) ;
#14145=VECTOR ( 'NONE', #7216, 1000.000000000000000 ) ;
#14177=DIRECTION ( 'NONE',  ( -0.000000000000000000, -0.000000000000000000, 1.000000000000000000 ) ) ;
#14198=EDGE_CURVE ( 'NONE', #11965, #7334, #2268, .T. ) ;
#14212=EDGE_CURVE ( 'NONE', #5643, #7514, #13332, .T. ) ;
#14221=CARTESIAN_POINT ( 'NONE',  ( 0.000000000000000000, 0.000000000000000000, 200.0000000000000000 ) ) ;
#14252=AXIS2_PLACEMENT_3D ( 'NONE', #1346, #11372, #11306 ) ;
#14278=VECTOR ( 'NONE', #7164, 1000.000000000000000 ) ;
#14293=ORIENTED_EDGE ( 'NONE', *, *, #13935, .F. ) ;
#14390=COLOUR_RGB('Light Blue',0.38,0.62,0.78);
#14391=FILL_AREA_STYLE_COLOUR('',#14390);
#14392=FILL_AREA_STYLE('',(#14391));
#14393=SURFACE_STYLE_FILL_AREA(#14392);
#14394=SURFACE_SIDE_STYLE('',(#14393));
#14395=SURFACE_STYLE_USAGE(.BOTH.,#14394);
#14396=PRESENTATION_STYLE_ASSIGNMENT((#14395));
ENDSEC;
END-ISO-10303-21;
